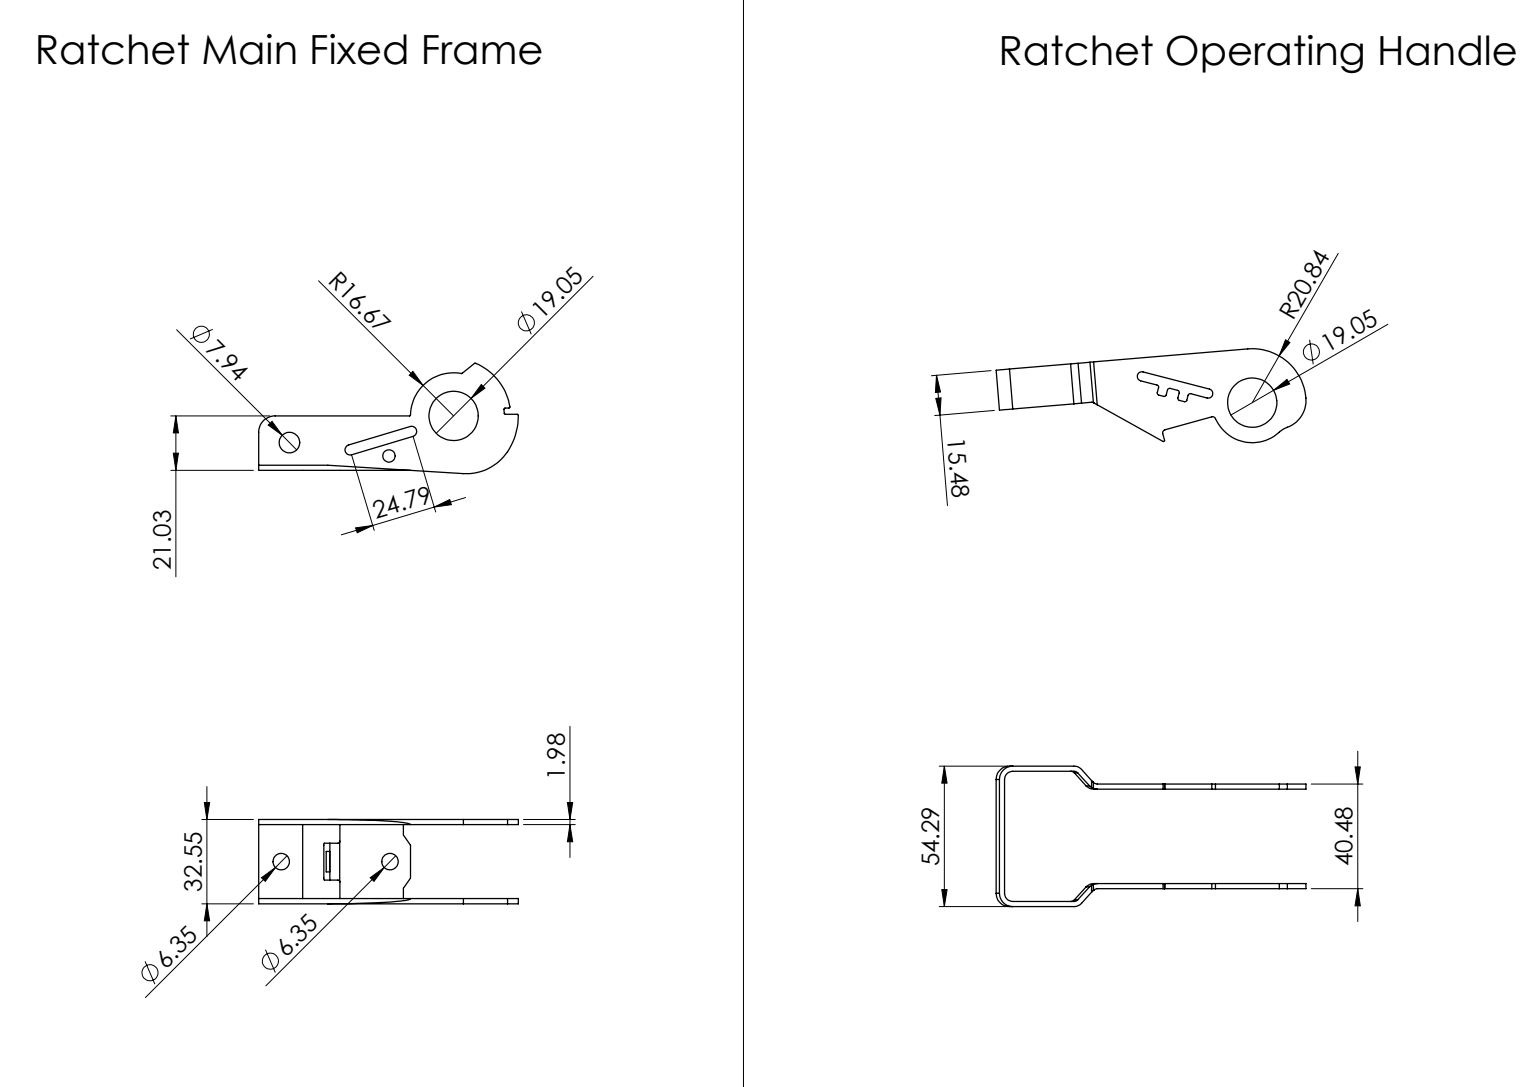
ISO-10303-21;
HEADER;
FILE_DESCRIPTION (('STEP AP214'),
    '1' );
FILE_NAME ('Ratchet Main Fixed Frame.step',
    '2026-10-09T14:10:49',
    ( '' ),
    ( '' ),
    'SwSTEP 2.0',
    'SolidWorks 2026',
    '' );
FILE_SCHEMA (( 'AUTOMOTIVE_DESIGN' ));
ENDSEC;

DATA;
#8=CARTESIAN_POINT ( 'NONE',  ( -23.01875000000000071, 1.984375000000000000, -3.968750000000000000 ) ) ;
#9=ADVANCED_FACE ( 'NONE', ( #16944, #16633 ), #1476, .F. ) ;
#15=CARTESIAN_POINT ( 'NONE',  ( -17.46249999999999858, 1.984375000000000000, 0.000000000000000000 ) ) ;
#18=CARTESIAN_POINT ( 'NONE',  ( 49.81956284419040060, 0.000000000000000000, 11.98436472153758103 ) ) ;
#22=VECTOR ( 'NONE', #6155, 999.9999999999998863 ) ;
#23=ORIENTED_EDGE ( 'NONE', *, *, #18650, .T. ) ;
#35=CARTESIAN_POINT ( 'NONE',  ( -29.36874999999999858, 2.380615000000000148, 8.335010000000000474 ) ) ;
#46=CIRCLE ( 'NONE', #17730, 1.984374999999999112 ) ;
#65=DIRECTION ( 'NONE',  ( 0.000000000000000000, 0.000000000000000000, -1.000000000000000000 ) ) ;
#67=AXIS2_PLACEMENT_3D ( 'NONE', #9052, #15829, #7402 ) ;
#70=ORIENTED_EDGE ( 'NONE', *, *, #12967, .F. ) ;
#71=AXIS2_PLACEMENT_3D ( 'NONE', #14766, #21802, #18271 ) ;
#74=PLANE ( 'NONE',  #18206 ) ;
#78=VECTOR ( 'NONE', #17853, 1000.000000000000227 ) ;
#94=AXIS2_PLACEMENT_3D ( 'NONE', #5064, #16687, #13274 ) ;
#104=CYLINDRICAL_SURFACE ( 'NONE', #7585, 0.3962400000000010358 ) ;
#109=CARTESIAN_POINT ( 'NONE',  ( 46.03750000000000142, 0.000000000000000000, -10.31874999999999964 ) ) ;
#117=CARTESIAN_POINT ( 'NONE',  ( 36.51250000000000284, 30.56064500000000095, -10.31875000000000142 ) ) ;
#120=EDGE_LOOP ( 'NONE', ( #10937, #5548, #3135, #2897 ) ) ;
#125=PLANE ( 'NONE',  #13958 ) ;
#133=DIRECTION ( 'NONE',  ( -0.9980811434661737147, 0.000000000000000000, -0.06191955310929838502 ) ) ;
#138=VERTEX_POINT ( 'NONE', #587 ) ;
#141=DIRECTION ( 'NONE',  ( 0.000000000000000000, 1.000000000000000000, 0.000000000000000000 ) ) ;
#150=DIRECTION ( 'NONE',  ( 0.000000000000000000, -1.000000000000000000, 0.000000000000000000 ) ) ;
#154=ORIENTED_EDGE ( 'NONE', *, *, #19245, .T. ) ;
#161=VECTOR ( 'NONE', #4886, 1000.000000000000227 ) ;
#162=LINE ( 'NONE', #18727, #15361 ) ;
#176=ORIENTED_EDGE ( 'NONE', *, *, #8308, .T. ) ;
#197=ORIENTED_EDGE ( 'NONE', *, *, #8367, .F. ) ;
#198=ORIENTED_EDGE ( 'NONE', *, *, #7883, .F. ) ;
#205=CARTESIAN_POINT ( 'NONE',  ( 29.36874999999999858, 0.000000000000000000, 10.71562499999999929 ) ) ;
#206=EDGE_LOOP ( 'NONE', ( #18423, #5151, #18532, #223 ) ) ;
#209=ORIENTED_EDGE ( 'NONE', *, *, #16573, .T. ) ;
#214=DIRECTION ( 'NONE',  ( 0.000000000000000000, 1.000000000000000000, 0.000000000000000000 ) ) ;
#218=VERTEX_POINT ( 'NONE', #12980 ) ;
#223=ORIENTED_EDGE ( 'NONE', *, *, #6828, .F. ) ;
#228=ORIENTED_EDGE ( 'NONE', *, *, #15345, .F. ) ;
#238=CARTESIAN_POINT ( 'NONE',  ( 54.11611804786240043, 30.56064500000000095, -30.58983753981140197 ) ) ;
#239=AXIS2_PLACEMENT_3D ( 'NONE', #18075, #4699, #2934 ) ;
#243=DIRECTION ( 'NONE',  ( -0.1831666983863990128, 0.000000000000000000, 0.9830818687180767901 ) ) ;
#259=LINE ( 'NONE', #5449, #10897 ) ;
#271=DIRECTION ( 'NONE',  ( 0.000000000000000000, 1.000000000000000000, 0.000000000000000000 ) ) ;
#280=DIRECTION ( 'NONE',  ( 0.000000000000000000, 1.000000000000000000, 0.000000000000000000 ) ) ;
#281=ORIENTED_EDGE ( 'NONE', *, *, #11678, .T. ) ;
#289=EDGE_CURVE ( 'NONE', #5674, #3944, #16188, .T. ) ;
#290=CARTESIAN_POINT ( 'NONE',  ( 6.016625000000000334, 1.984375000000000000, 2.794000000000000039 ) ) ;
#291=CARTESIAN_POINT ( 'NONE',  ( -29.36874999999999858, 9.129395000000000593, 0.000000000000000000 ) ) ;
#295=CARTESIAN_POINT ( 'NONE',  ( 18.65312499999999929, 0.000000000000000000, 5.159374999999999822 ) ) ;
#301=DIRECTION ( 'NONE',  ( 0.000000000000000000, 1.000000000000000000, 0.000000000000000000 ) ) ;
#311=EDGE_CURVE ( 'NONE', #1101, #20045, #18407, .T. ) ;
#313=DIRECTION ( 'NONE',  ( 0.000000000000000000, -1.000000000000000000, 0.000000000000000000 ) ) ;
#316=EDGE_CURVE ( 'NONE', #18861, #19124, #21090, .T. ) ;
#319=EDGE_CURVE ( 'NONE', #2537, #9809, #10285, .T. ) ;
#322=CARTESIAN_POINT ( 'NONE',  ( 1.954387715434429795, -42.42568807200000691, 6.745605000000000295 ) ) ;
#323=CARTESIAN_POINT ( 'NONE',  ( 67.40134256979101224, 0.000000000000000000, -13.70358117861468017 ) ) ;
#326=ORIENTED_EDGE ( 'NONE', *, *, #979, .T. ) ;
#354=DIRECTION ( 'NONE',  ( -0.9579671649362033747, 0.000000000000000000, 0.2868778675745011220 ) ) ;
#364=LINE ( 'NONE', #8871, #4198 ) ;
#377=VECTOR ( 'NONE', #1528, 1000.000000000000000 ) ;
#391=LINE ( 'NONE', #12123, #16283 ) ;
#395=VERTEX_POINT ( 'NONE', #5841 ) ;
#411=VECTOR ( 'NONE', #16269, 1000.000000000000114 ) ;
#417=ORIENTED_EDGE ( 'NONE', *, *, #10498, .T. ) ;
#418=EDGE_LOOP ( 'NONE', ( #15231, #7592, #4547, #16029 ) ) ;
#436=VECTOR ( 'NONE', #9326, 1000.000000000000000 ) ;
#442=DIRECTION ( 'NONE',  ( -0.2868778675745010664, 0.000000000000000000, -0.9579671649362032637 ) ) ;
#447=CARTESIAN_POINT ( 'NONE',  ( -29.36874999999999858, 0.000000000000000000, -3.968750000000000000 ) ) ;
#468=EDGE_CURVE ( 'NONE', #14260, #16212, #12495, .T. ) ;
#501=EDGE_LOOP ( 'NONE', ( #16352, #7920, #20206, #7975 ) ) ;
#505=ORIENTED_EDGE ( 'NONE', *, *, #10172, .T. ) ;
#507=DIRECTION ( 'NONE',  ( 0.000000000000000000, -1.000000000000000000, 0.000000000000000000 ) ) ;
#511=ORIENTED_EDGE ( 'NONE', *, *, #13513, .F. ) ;
#516=ORIENTED_EDGE ( 'NONE', *, *, #17729, .F. ) ;
#518=AXIS2_PLACEMENT_3D ( 'NONE', #7879, #21361, #11096 ) ;
#528=CARTESIAN_POINT ( 'NONE',  ( 46.03750000000000142, 0.000000000000000000, -10.31874999999999964 ) ) ;
#554=CIRCLE ( 'NONE', #4091, 0.3962399999999999811 ) ;
#564=EDGE_LOOP ( 'NONE', ( #7716, #9815, #9669, #1208 ) ) ;
#572=PLANE ( 'NONE',  #16036 ) ;
#581=CARTESIAN_POINT ( 'NONE',  ( 29.19635173153840313, 32.54502000000000095, -6.218966092919240296 ) ) ;
#582=FACE_BOUND ( 'NONE', #7037, .T. ) ;
#587=CARTESIAN_POINT ( 'NONE',  ( 49.41235866845560309, 32.54502000000000095, -26.78690084448080100 ) ) ;
#622=CARTESIAN_POINT ( 'NONE',  ( 65.90927232300019512, 0.000000000000000000, -13.30734117861468135 ) ) ;
#628=ORIENTED_EDGE ( 'NONE', *, *, #11808, .F. ) ;
#629=CYLINDRICAL_SURFACE ( 'NONE', #3313, 0.3962399999999990929 ) ;
#630=CARTESIAN_POINT ( 'NONE',  ( 1.952969610814715207, 8.739187247087119914, 8.731249999999999289 ) ) ;
#632=ORIENTED_EDGE ( 'NONE', *, *, #7507, .T. ) ;
#641=EDGE_CURVE ( 'NONE', #1856, #20988, #8151, .T. ) ;
#642=ORIENTED_EDGE ( 'NONE', *, *, #17287, .T. ) ;
#646=CARTESIAN_POINT ( 'NONE',  ( 18.74375446079810104, 0.5063334429457699848, 10.05646519131946093 ) ) ;
#648=DIRECTION ( 'NONE',  ( 0.000000000000000000, -1.000000000000000000, 0.000000000000000000 ) ) ;
#655=DIRECTION ( 'NONE',  ( 0.000000000000000000, 1.000000000000000000, 0.000000000000000000 ) ) ;
#656=DIRECTION ( 'NONE',  ( 0.000000000000000000, -1.000000000000000000, 0.000000000000000000 ) ) ;
#658=ORIENTED_EDGE ( 'NONE', *, *, #14396, .F. ) ;
#664=EDGE_LOOP ( 'NONE', ( #18136, #17984, #7800, #6958 ) ) ;
#665=EDGE_CURVE ( 'NONE', #14162, #4933, #12805, .T. ) ;
#677=CYLINDRICAL_SURFACE ( 'NONE', #11422, 0.3962400000000008138 ) ;
#691=EDGE_CURVE ( 'NONE', #3431, #18275, #1843, .T. ) ;
#695=ORIENTED_EDGE ( 'NONE', *, *, #7242, .F. ) ;
#705=EDGE_CURVE ( 'NONE', #1101, #3875, #6823, .T. ) ;
#708=LINE ( 'NONE', #15884, #14164 ) ;
#710=EDGE_LOOP ( 'NONE', ( #9718, #14667, #1796, #5850, #15920 ) ) ;
#717=LINE ( 'NONE', #12670, #3287 ) ;
#726=CARTESIAN_POINT ( 'NONE',  ( 1.268730000000000135, 9.129395000000000593, 8.609509071587499562 ) ) ;
#729=CIRCLE ( 'NONE', #7799, 2.381250000000001421 ) ;
#731=EDGE_LOOP ( 'NONE', ( #7711, #2068 ) ) ;
#733=AXIS2_PLACEMENT_3D ( 'NONE', #2522, #9471, #14263 ) ;
#735=EDGE_CURVE ( 'NONE', #12688, #16536, #11693, .T. ) ;
#738=LINE ( 'NONE', #19310, #21439 ) ;
#739=VECTOR ( 'NONE', #11879, 1000.000000000000000 ) ;
#743=ADVANCED_FACE ( 'NONE', ( #9913 ), #18750, .T. ) ;
#757=CARTESIAN_POINT ( 'NONE',  ( 6.472296726610020201, 0.08030987734106199982, 9.295161179239141092 ) ) ;
#764=EDGE_CURVE ( 'NONE', #7013, #13795, #15358, .T. ) ;
#765=ORIENTED_EDGE ( 'NONE', *, *, #8954, .T. ) ;
#768=DIRECTION ( 'NONE',  ( 0.2868778675745004558, 0.000000000000000000, 0.9579671649362035968 ) ) ;
#771=EDGE_LOOP ( 'NONE', ( #6023, #8487, #4066, #14596 ) ) ;
#772=ORIENTED_EDGE ( 'NONE', *, *, #5768, .T. ) ;
#777=VERTEX_POINT ( 'NONE', #19975 ) ;
#793=VECTOR ( 'NONE', #3732, 1000.000000000000114 ) ;
#796=DIRECTION ( 'NONE',  ( 0.000000000000000000, 1.000000000000000000, 0.000000000000000000 ) ) ;
#798=CARTESIAN_POINT ( 'NONE',  ( 6.585898268469219552, 30.56064500000000095, 4.694966092919240275 ) ) ;
#812=DIRECTION ( 'NONE',  ( 0.000000000000000000, 1.000000000000000000, 0.000000000000000000 ) ) ;
#817=AXIS2_PLACEMENT_3D ( 'NONE', #3190, #18327, #3407 ) ;
#818=CARTESIAN_POINT ( 'NONE',  ( -2.028188046367890074, 9.924415000000001541, 0.3682158094503220069 ) ) ;
#825=VECTOR ( 'NONE', #16124, 1000.000000000000227 ) ;
#827=DIRECTION ( 'NONE',  ( 0.000000000000000000, 1.000000000000000000, 0.000000000000000000 ) ) ;
#833=CARTESIAN_POINT ( 'NONE',  ( 26.59062499999999929, 2.380615000000000148, 8.731249999999999289 ) ) ;
#840=CARTESIAN_POINT ( 'NONE',  ( 26.59062499999999929, 5.953125000000000000, 10.71562499999999929 ) ) ;
#843=EDGE_CURVE ( 'NONE', #5953, #16263, #20185, .T. ) ;
#852=CIRCLE ( 'NONE', #12513, 0.3962399999999990929 ) ;
#854=EDGE_LOOP ( 'NONE', ( #772, #16081, #18567, #4619, #13382, #13035, #9205, #19390, #3885, #9519, #20998, #18124, #9666, #2739, #11741, #2851, #8488, #10820, #3221, #4979, #18354 ) ) ;
#857=AXIS2_PLACEMENT_3D ( 'NONE', #12113, #15668, #1410 ) ;
#860=FACE_OUTER_BOUND ( 'NONE', #15123, .T. ) ;
#873=CARTESIAN_POINT ( 'NONE',  ( 11.57071721368057915, 0.2046444788096904999, 9.611460029477360223 ) ) ;
#894=DIRECTION ( 'NONE',  ( 0.2868778675745010664, 0.000000000000000000, 0.9579671649362032637 ) ) ;
#896=EDGE_CURVE ( 'NONE', #10916, #13402, #20547, .T. ) ;
#908=CARTESIAN_POINT ( 'NONE',  ( 1.336191582698512681, 23.41816499999998769, 10.66779613908654056 ) ) ;
#915=CARTESIAN_POINT ( 'NONE',  ( 29.35287372532640049, 1.909660849011530104, 10.71464187463071838 ) ) ;
#922=ADVANCED_FACE ( 'NONE', ( #2286 ), #10909, .F. ) ;
#937=DIRECTION ( 'NONE',  ( 0.000000000000000000, 0.000000000000000000, 1.000000000000000000 ) ) ;
#943=EDGE_CURVE ( 'NONE', #17008, #1261, #5484, .T. ) ;
#955=DIRECTION ( 'NONE',  ( 1.000000000000000000, 0.000000000000000000, 0.000000000000000000 ) ) ;
#958=CARTESIAN_POINT ( 'NONE',  ( 65.90927232300019512, 32.54502000000000095, -13.30734117861468135 ) ) ;
#966=VERTEX_POINT ( 'NONE', #17658 ) ;
#971=CARTESIAN_POINT ( 'NONE',  ( 2.063750000000000195, 1.984375000000000000, -16.49278420930464861 ) ) ;
#974=ORIENTED_EDGE ( 'NONE', *, *, #1086, .T. ) ;
#978=CARTESIAN_POINT ( 'NONE',  ( -29.36874999999999858, 2.380615000000000148, 8.731249999999999289 ) ) ;
#979=EDGE_CURVE ( 'NONE', #12825, #9462, #12474, .T. ) ;
#986=ORIENTED_EDGE ( 'NONE', *, *, #17962, .F. ) ;
#1004=CARTESIAN_POINT ( 'NONE',  ( 2.063750000000000195, 24.21318500000000284, 10.71562499999999929 ) ) ;
#1007=DIRECTION ( 'NONE',  ( 1.000000000000000000, 0.000000000000000000, 0.000000000000000000 ) ) ;
#1012=PRODUCT_DEFINITION ( 'UNKNOWN', '', #20389, #10115 ) ;
#1016=CARTESIAN_POINT ( 'NONE',  ( 26.96090640492720425, 1.228048945539309766, 10.56624576331076071 ) ) ;
#1019=DIRECTION ( 'NONE',  ( -0.9966381950048638361, 0.000000000000000000, 0.08192867786951606168 ) ) ;
#1025=ORIENTED_EDGE ( 'NONE', *, *, #19522, .F. ) ;
#1027=DIRECTION ( 'NONE',  ( 1.000000000000000000, 0.000000000000000000, 0.000000000000000000 ) ) ;
#1031=FACE_OUTER_BOUND ( 'NONE', #17461, .T. ) ;
#1040=ORIENTED_EDGE ( 'NONE', *, *, #6973, .F. ) ;
#1051=CIRCLE ( 'NONE', #4594, 0.3962399999999999811 ) ;
#1058=( GEOMETRIC_REPRESENTATION_CONTEXT ( 3 ) GLOBAL_UNCERTAINTY_ASSIGNED_CONTEXT ( ( #18944 ) ) GLOBAL_UNIT_ASSIGNED_CONTEXT ( ( #20231, #6550, #3348 ) ) REPRESENTATION_CONTEXT ( 'NONE', 'WORKASPACE' ) );
#1061=CARTESIAN_POINT ( 'NONE',  ( 70.64340948846358970, 32.54502000000000095, -10.93409647675949969 ) ) ;
#1062=ORIENTED_EDGE ( 'NONE', *, *, #13513, .T. ) ;
#1067=ORIENTED_EDGE ( 'NONE', *, *, #1108, .F. ) ;
#1076=ORIENTED_EDGE ( 'NONE', *, *, #468, .T. ) ;
#1082=AXIS2_PLACEMENT_3D ( 'NONE', #19728, #13446, #18513 ) ;
#1084=CARTESIAN_POINT ( 'NONE',  ( 46.03750000000000142, 32.54502000000000095, -10.31874999999999964 ) ) ;
#1086=EDGE_CURVE ( 'NONE', #10374, #6204, #17753, .T. ) ;
#1087=AXIS2_PLACEMENT_3D ( 'NONE', #11496, #6526, #8379 ) ;
#1094=FACE_OUTER_BOUND ( 'NONE', #16465, .T. ) ;
#1101=VERTEX_POINT ( 'NONE', #21702 ) ;
#1107=AXIS2_PLACEMENT_3D ( 'NONE', #8605, #15486, #8489 ) ;
#1108=EDGE_CURVE ( 'NONE', #9462, #16780, #13415, .T. ) ;
#1111=DIRECTION ( 'NONE',  ( -0.9579671649362032637, 0.000000000000000000, 0.2868778675745010664 ) ) ;
#1120=DIRECTION ( 'NONE',  ( 0.000000000000000000, 0.000000000000000000, 1.000000000000000000 ) ) ;
#1127=CARTESIAN_POINT ( 'NONE',  ( 28.31895198753520049, 1.479004908355108006, 10.65049700491969986 ) ) ;
#1132=DIRECTION ( 'NONE',  ( 1.000000000000000000, 0.000000000000000000, 0.000000000000000000 ) ) ;
#1135=DIRECTION ( 'NONE',  ( 0.000000000000000000, 1.000000000000000000, 0.000000000000000000 ) ) ;
#1139=AXIS2_PLACEMENT_3D ( 'NONE', #15940, #16049, #10935 ) ;
#1140=CYLINDRICAL_SURFACE ( 'NONE', #6685, 22.02656249999999361 ) ;
#1142=CARTESIAN_POINT ( 'NONE',  ( 6.016625000000000334, 32.54502000000000095, 2.794000000000000039 ) ) ;
#1145=CIRCLE ( 'NONE', #3270, 6.349999999999999645 ) ;
#1156=VECTOR ( 'NONE', #3402, 1000.000000000000000 ) ;
#1161=DIRECTION ( 'NONE',  ( 0.000000000000000000, 1.000000000000000000, 0.000000000000000000 ) ) ;
#1162=ORIENTED_EDGE ( 'NONE', *, *, #15592, .F. ) ;
#1164=EDGE_LOOP ( 'NONE', ( #7263, #18315, #20283, #12931 ) ) ;
#1168=ADVANCED_FACE ( 'NONE', ( #11530 ), #8094, .T. ) ;
#1171=ORIENTED_EDGE ( 'NONE', *, *, #15592, .T. ) ;
#1179=ORIENTED_EDGE ( 'NONE', *, *, #6973, .T. ) ;
#1182=ORIENTED_EDGE ( 'NONE', *, *, #6183, .F. ) ;
#1186=DIRECTION ( 'NONE',  ( 0.000000000000000000, -1.000000000000000000, 0.000000000000000000 ) ) ;
#1187=EDGE_LOOP ( 'NONE', ( #19885, #4119, #17539, #10765 ) ) ;
#1195=VECTOR ( 'NONE', #7827, 999.9999999999998863 ) ;
#1202=VERTEX_POINT ( 'NONE', #19816 ) ;
#1204=CARTESIAN_POINT ( 'NONE',  ( 26.59062499871549790, 1.984216250000009785, 10.71562498306123956 ) ) ;
#1208=ORIENTED_EDGE ( 'NONE', *, *, #20286, .F. ) ;
#1212=DIRECTION ( 'NONE',  ( 1.000000000000000000, 0.000000000000000000, 0.000000000000000000 ) ) ;
#1215=EDGE_LOOP ( 'NONE', ( #5293, #9550, #511, #6847 ) ) ;
#1239=DIRECTION ( 'NONE',  ( -0.7776383362760926898, 0.000000000000000000, 0.6287118719681938916 ) ) ;
#1243=DIRECTION ( 'NONE',  ( 1.000000000000000000, 0.000000000000000000, 0.000000000000000000 ) ) ;
#1249=DIRECTION ( 'NONE',  ( 0.000000000000000000, 1.000000000000000000, 0.000000000000000000 ) ) ;
#1252=CARTESIAN_POINT ( 'NONE',  ( -3.929154139288399961, 22.62314500000000095, 0.9374890779182719625 ) ) ;
#1256=EDGE_LOOP ( 'NONE', ( #8055, #5991, #15134, #11048, #17890, #4299 ) ) ;
#1260=AXIS2_PLACEMENT_3D ( 'NONE', #13322, #14664, #16739 ) ;
#1261=VERTEX_POINT ( 'NONE', #10524 ) ;
#1266=VERTEX_POINT ( 'NONE', #12086 ) ;
#1286=CARTESIAN_POINT ( 'NONE',  ( 21.03437500000000071, 30.56064500000000095, 5.159374999999999822 ) ) ;
#1302=CARTESIAN_POINT ( 'NONE',  ( 71.03963378001139972, 32.54502000000000095, -10.54138470677948014 ) ) ;
#1307=CARTESIAN_POINT ( 'NONE',  ( 201.9384738932629944, 1.984375000000000000, 10.71562489836746046 ) ) ;
#1311=EDGE_CURVE ( 'NONE', #7810, #19275, #7545, .T. ) ;
#1319=DIRECTION ( 'NONE',  ( 0.2868778675745004558, 0.000000000000000000, 0.9579671649362035968 ) ) ;
#1331=CARTESIAN_POINT ( 'NONE',  ( 1.603561069792159621, 23.48871702854725996, 10.70056859876313382 ) ) ;
#1335=ORIENTED_EDGE ( 'NONE', *, *, #3563, .F. ) ;
#1344=FACE_OUTER_BOUND ( 'NONE', #19634, .T. ) ;
#1346=DIRECTION ( 'NONE',  ( 0.000000000000000000, -1.000000000000000000, 0.000000000000000000 ) ) ;
#1349=AXIS2_PLACEMENT_3D ( 'NONE', #35, #13658, #3583 ) ;
#1356=VERTEX_POINT ( 'NONE', #2346 ) ;
#1378=CIRCLE ( 'NONE', #4216, 0.3962399999999988154 ) ;
#1385=ADVANCED_FACE ( 'NONE', ( #4114 ), #10856, .F. ) ;
#1386=ADVANCED_FACE ( 'NONE', ( #17394 ), #7323, .T. ) ;
#1389=CARTESIAN_POINT ( 'NONE',  ( 46.03750000000000142, 0.000000000000000000, -10.31874999999999964 ) ) ;
#1394=CARTESIAN_POINT ( 'NONE',  ( 55.56250000000000000, 30.56064500000000095, -10.31874999999999964 ) ) ;
#1395=ORIENTED_EDGE ( 'NONE', *, *, #4129, .T. ) ;
#1399=ORIENTED_EDGE ( 'NONE', *, *, #12967, .T. ) ;
#1402=VERTEX_POINT ( 'NONE', #798 ) ;
#1410=DIRECTION ( 'NONE',  ( 1.000000000000000000, 0.000000000000000000, 0.000000000000000000 ) ) ;
#1413=EDGE_CURVE ( 'NONE', #10320, #7268, #19359, .T. ) ;
#1417=CARTESIAN_POINT ( 'NONE',  ( 46.03750000000000142, 30.56064500000000095, -10.31874999999999964 ) ) ;
#1418=FACE_OUTER_BOUND ( 'NONE', #9038, .T. ) ;
#1420=ORIENTED_EDGE ( 'NONE', *, *, #5878, .F. ) ;
#1421=ORIENTED_EDGE ( 'NONE', *, *, #14670, .T. ) ;
#1424=CARTESIAN_POINT ( 'NONE',  ( 67.40134256979101224, 32.54502000000000095, -13.30734117861468135 ) ) ;
#1427=CARTESIAN_POINT ( 'NONE',  ( 26.59062499999999929, 5.953125000000000000, 8.731249999999999289 ) ) ;
#1428=AXIS2_PLACEMENT_3D ( 'NONE', #20915, #20685, #5542 ) ;
#1432=EDGE_CURVE ( 'NONE', #6164, #7181, #16178, .T. ) ;
#1433=VECTOR ( 'NONE', #5276, 1000.000000000000000 ) ;
#1441=DIRECTION ( 'NONE',  ( 0.9966381950048638361, 0.000000000000000000, -0.08192867786951699149 ) ) ;
#1445=EDGE_LOOP ( 'NONE', ( #18109, #19711, #10943, #9247 ) ) ;
#1449=VERTEX_POINT ( 'NONE', #21235 ) ;
#1451=VECTOR ( 'NONE', #4832, 1000.000000000000000 ) ;
#1453=LINE ( 'NONE', #21355, #13072 ) ;
#1455=AXIS2_PLACEMENT_3D ( 'NONE', #16323, #11654, #19616 ) ;
#1458=DIRECTION ( 'NONE',  ( 0.2868778675745011220, 0.000000000000000000, 0.9579671649362033747 ) ) ;
#1469=CARTESIAN_POINT ( 'NONE',  ( -2.256261688646920227, 9.924415000000001541, -0.3933872460174320240 ) ) ;
#1476=PLANE ( 'NONE',  #5340 ) ;
#1486=DIRECTION ( 'NONE',  ( -0.9579671649362032637, 0.000000000000000000, 0.2868778675745010664 ) ) ;
#1498=FACE_OUTER_BOUND ( 'NONE', #6214, .T. ) ;
#1502=CARTESIAN_POINT ( 'NONE',  ( 65.64431122251959039, 0.000000000000000000, -11.29787305743958115 ) ) ;
#1503=EDGE_LOOP ( 'NONE', ( #2825, #2613, #15196, #20000 ) ) ;
#1522=CARTESIAN_POINT ( 'NONE',  ( 54.11611804786240043, 1.984375000000000000, -30.58983753981140197 ) ) ;
#1523=DIRECTION ( 'NONE',  ( 0.000000000000000000, 0.000000000000000000, -1.000000000000000000 ) ) ;
#1528=DIRECTION ( 'NONE',  ( 0.000000000000000000, 1.000000000000000000, 0.000000000000000000 ) ) ;
#1534=DIRECTION ( 'NONE',  ( 1.000000000000000000, 0.000000000000000000, 0.000000000000000000 ) ) ;
#1539=CARTESIAN_POINT ( 'NONE',  ( -12.30312499999999964, 30.56064500000000095, 8.731249999999999289 ) ) ;
#1543=EDGE_CURVE ( 'NONE', #10050, #7714, #3297, .T. ) ;
#1547=PLANE ( 'NONE',  #20270 ) ;
#1550=ORIENTED_EDGE ( 'NONE', *, *, #5921, .F. ) ;
#1552=AXIS2_PLACEMENT_3D ( 'NONE', #9619, #13292, #21231 ) ;
#1553=PLANE ( 'NONE',  #6412 ) ;
#1561=EDGE_CURVE ( 'NONE', #16780, #6164, #2753, .T. ) ;
#1572=DIRECTION ( 'NONE',  ( -0.7776383362760926898, 0.000000000000000000, 0.6287118719681938916 ) ) ;
#1576=DIRECTION ( 'NONE',  ( 0.000000000000000000, 1.000000000000000000, 0.000000000000000000 ) ) ;
#1589=CARTESIAN_POINT ( 'NONE',  ( 26.59062499999999929, 2.380615000000000148, 8.335010000000000474 ) ) ;
#1593=CARTESIAN_POINT ( 'NONE',  ( -29.36874999999999858, 30.16440499999999858, 8.731249999999999289 ) ) ;
#1626=EDGE_LOOP ( 'NONE', ( #16316, #15503, #7681, #7730 ) ) ;
#1629=CARTESIAN_POINT ( 'NONE',  ( 46.03750000000000142, 1.984375000000000000, -10.31874999999999964 ) ) ;
#1639=LINE ( 'NONE', #3320, #14876 ) ;
#1641=ORIENTED_EDGE ( 'NONE', *, *, #12188, .F. ) ;
#1644=EDGE_CURVE ( 'NONE', #11015, #3875, #17773, .T. ) ;
#1648=CARTESIAN_POINT ( 'NONE',  ( -4.157227781567939928, 9.129395000000000593, 0.1758860224507720060 ) ) ;
#1655=CARTESIAN_POINT ( 'NONE',  ( -17.46249999999999858, 30.56064500000000095, 0.000000000000000000 ) ) ;
#1659=ADVANCED_FACE ( 'NONE', ( #17113 ), #3627, .F. ) ;
#1668=CARTESIAN_POINT ( 'NONE',  ( 54.29867169743560140, 0.000000000000000000, -30.73743011777780154 ) ) ;
#1672=CARTESIAN_POINT ( 'NONE',  ( 28.97711086133420366, 32.54502000000000095, -10.71499000000000024 ) ) ;
#1683=DIRECTION ( 'NONE',  ( 0.000000000000000000, 1.000000000000000000, 0.000000000000000000 ) ) ;
#1684=DIRECTION ( 'NONE',  ( 1.000000000000000000, 0.000000000000000000, 0.000000000000000000 ) ) ;
#1686=CARTESIAN_POINT ( 'NONE',  ( 5.447351731530780228, 30.56064500000000095, 0.8930339070797439494 ) ) ;
#1694=CARTESIAN_POINT ( 'NONE',  ( 46.03750000000000142, 0.000000000000000000, -10.31874999999999964 ) ) ;
#1704=EDGE_CURVE ( 'NONE', #17862, #13475, #2935, .T. ) ;
#1709=ORIENTED_EDGE ( 'NONE', *, *, #4496, .T. ) ;
#1713=B_SPLINE_CURVE_WITH_KNOTS ( 'NONE', 3,
 ( #12498, #7513, #19221, #4190, #10495, #15718, #17682, #2534 ),
 .UNSPECIFIED., .F., .F.,
 ( 4, 2, 2, 4 ),
 ( 0.000000000000000000, 0.2499999999999987232, 0.4999999999999974465, 1.000000000000000000 ),
 .UNSPECIFIED. ) ;
#1714=VERTEX_POINT ( 'NONE', #6609 ) ;
#1728=AXIS2_PLACEMENT_3D ( 'NONE', #5068, #1959, #20517 ) ;
#1734=VECTOR ( 'NONE', #18310, 1000.000000000000114 ) ;
#1736=DIRECTION ( 'NONE',  ( 0.000000000000000000, 1.000000000000000000, 0.000000000000000000 ) ) ;
#1737=CARTESIAN_POINT ( 'NONE',  ( 46.03750000000000142, 32.54502000000000095, -10.31874999999999964 ) ) ;
#1739=LINE ( 'NONE', #5067, #13841 ) ;
#1747=ORIENTED_EDGE ( 'NONE', *, *, #6828, .T. ) ;
#1748=DIRECTION ( 'NONE',  ( 0.000000000000000000, 1.000000000000000000, 0.000000000000000000 ) ) ;
#1751=EDGE_CURVE ( 'NONE', #4180, #17367, #17419, .T. ) ;
#1752=DIRECTION ( 'NONE',  ( 0.9999603561554373243, 0.000000000000000000, -0.008904275236710241376 ) ) ;
#1753=CARTESIAN_POINT ( 'NONE',  ( 29.37324403177899868, 0.000000000000000000, -10.70578951775076071 ) ) ;
#1756=FACE_OUTER_BOUND ( 'NONE', #854, .T. ) ;
#1771=DIRECTION ( 'NONE',  ( 0.000000000000000000, 1.000000000000000000, 0.000000000000000000 ) ) ;
#1774=AXIS2_PLACEMENT_3D ( 'NONE', #10053, #8282, #6290 ) ;
#1776=FACE_OUTER_BOUND ( 'NONE', #9027, .T. ) ;
#1796=ORIENTED_EDGE ( 'NONE', *, *, #10074, .F. ) ;
#1798=CARTESIAN_POINT ( 'NONE',  ( 71.04062499999999147, 0.000000000000000000, -10.31874999999999964 ) ) ;
#1801=ORIENTED_EDGE ( 'NONE', *, *, #20190, .T. ) ;
#1825=CIRCLE ( 'NONE', #3243, 1.984374999999998890 ) ;
#1831=ORIENTED_EDGE ( 'NONE', *, *, #17908, .T. ) ;
#1838=ORIENTED_EDGE ( 'NONE', *, *, #10629, .F. ) ;
#1839=DIRECTION ( 'NONE',  ( 0.000000000000000000, 1.000000000000000000, 0.000000000000000000 ) ) ;
#1843=LINE ( 'NONE', #15037, #8191 ) ;
#1856=VERTEX_POINT ( 'NONE', #19308 ) ;
#1859=CARTESIAN_POINT ( 'NONE',  ( -29.36874999999999858, 0.000000000000000000, 8.731885000000000119 ) ) ;
#1871=ORIENTED_EDGE ( 'NONE', *, *, #10172, .F. ) ;
#1876=VERTEX_POINT ( 'NONE', #4170 ) ;
#1882=ORIENTED_EDGE ( 'NONE', *, *, #3188, .T. ) ;
#1891=EDGE_CURVE ( 'NONE', #21568, #12583, #7167, .T. ) ;
#1893=CIRCLE ( 'NONE', #8262, 3.175000000000000711 ) ;
#1895=CARTESIAN_POINT ( 'NONE',  ( -20.63749999999999929, 16.27314499999999953, 8.731249999999999289 ) ) ;
#1898=DIRECTION ( 'NONE',  ( 0.000000000000000000, -1.000000000000000000, 0.000000000000000000 ) ) ;
#1900=AXIS2_PLACEMENT_3D ( 'NONE', #18001, #14482, #6058 ) ;
#1908=CARTESIAN_POINT ( 'NONE',  ( 6.585898268469219552, 1.984375000000000000, 4.694966092919240275 ) ) ;
#1917=ORIENTED_EDGE ( 'NONE', *, *, #6375, .F. ) ;
#1931=ORIENTED_EDGE ( 'NONE', *, *, #21706, .T. ) ;
#1954=ORIENTED_EDGE ( 'NONE', *, *, #11915, .F. ) ;
#1958=CARTESIAN_POINT ( 'NONE',  ( 26.59062499999999929, 2.380615000000000148, 8.731249999999999289 ) ) ;
#1959=DIRECTION ( 'NONE',  ( 0.000000000000000000, 1.000000000000000000, 0.000000000000000000 ) ) ;
#1972=LINE ( 'NONE', #15490, #17384 ) ;
#1975=ADVANCED_FACE ( 'NONE', ( #3738 ), #629, .F. ) ;
#1977=DIRECTION ( 'NONE',  ( 0.000000000000000000, 0.000000000000000000, -1.000000000000000000 ) ) ;
#2020=VERTEX_POINT ( 'NONE', #20740 ) ;
#2027=DIRECTION ( 'NONE',  ( 1.000000000000000000, 0.000000000000000000, 0.000000000000000000 ) ) ;
#2032=ORIENTED_EDGE ( 'NONE', *, *, #19528, .F. ) ;
#2034=DIRECTION ( 'NONE',  ( 0.000000000000000000, -1.000000000000000000, 0.000000000000000000 ) ) ;
#2047=EDGE_CURVE ( 'NONE', #18768, #2822, #14695, .T. ) ;
#2051=CARTESIAN_POINT ( 'NONE',  ( -29.36874999999999858, 30.56128000000000000, 10.71562499999999929 ) ) ;
#2053=CARTESIAN_POINT ( 'NONE',  ( 0.02083138522551555155, 12.30439499999999953, 7.210477125664100484 ) ) ;
#2055=CARTESIAN_POINT ( 'NONE',  ( 1.402240371799016394, 9.120973559619994120, 10.67764259629631951 ) ) ;
#2063=ORIENTED_EDGE ( 'NONE', *, *, #15564, .F. ) ;
#2068=ORIENTED_EDGE ( 'NONE', *, *, #11302, .T. ) ;
#2076=CIRCLE ( 'NONE', #7372, 3.968750000000000000 ) ;
#2079=DIRECTION ( 'NONE',  ( 0.000000000000000000, 0.000000000000000000, -1.000000000000000000 ) ) ;
#2081=CARTESIAN_POINT ( 'NONE',  ( 17.77223365658175069, 0.4543760498246959822, 9.996193404372801794 ) ) ;
#2082=CIRCLE ( 'NONE', #15531, 0.7950200000000000600 ) ;
#2087=LINE ( 'NONE', #20216, #11922 ) ;
#2089=CARTESIAN_POINT ( 'NONE',  ( -3.246390552019219999, 12.30439499999999953, 3.217431771123079987 ) ) ;
#2091=LINE ( 'NONE', #10831, #6773 ) ;
#2092=ORIENTED_EDGE ( 'NONE', *, *, #11972, .F. ) ;
#2108=EDGE_CURVE ( 'NONE', #10320, #2958, #18819, .T. ) ;
#2113=DIRECTION ( 'NONE',  ( 0.000000000000000000, 1.000000000000000000, 0.000000000000000000 ) ) ;
#2122=VECTOR ( 'NONE', #827, 1000.000000000000000 ) ;
#2127=AXIS2_PLACEMENT_3D ( 'NONE', #12879, #11421, #1243 ) ;
#2137=ORIENTED_EDGE ( 'NONE', *, *, #16907, .F. ) ;
#2146=CARTESIAN_POINT ( 'NONE',  ( 65.51436440461340283, 0.000000000000000000, -12.87863775929475985 ) ) ;
#2151=EDGE_LOOP ( 'NONE', ( #4488, #19389, #2830, #5520 ) ) ;
#2159=CIRCLE ( 'NONE', #15957, 0.7950199999999998379 ) ;
#2165=CIRCLE ( 'NONE', #14549, 1.983739999999999393 ) ;
#2167=ORIENTED_EDGE ( 'NONE', *, *, #18913, .F. ) ;
#2173=CARTESIAN_POINT ( 'NONE',  ( 1.603642987080700744, 9.058787236897966721, 10.70057449157679663 ) ) ;
#2178=CARTESIAN_POINT ( 'NONE',  ( 71.03963378001139972, 0.000000000000000000, -10.54138470677948014 ) ) ;
#2179=CARTESIAN_POINT ( 'NONE',  ( 26.59062499999999929, 30.56064500000000095, 8.335010000000000474 ) ) ;
#2212=VERTEX_POINT ( 'NONE', #17883 ) ;
#2217=VERTEX_POINT ( 'NONE', #21294 ) ;
#2219=DIRECTION ( 'NONE',  ( 0.000000000000000000, 1.000000000000000000, 0.000000000000000000 ) ) ;
#2221=CIRCLE ( 'NONE', #3289, 0.3962399999999997591 ) ;
#2226=CARTESIAN_POINT ( 'NONE',  ( 1.954387715434429795, 8.736780638212259475, 10.71562499999999929 ) ) ;
#2228=ADVANCED_FACE ( 'NONE', ( #5563 ), #3924, .T. ) ;
#2234=AXIS2_PLACEMENT_3D ( 'NONE', #14022, #2275, #17644 ) ;
#2236=CYLINDRICAL_SURFACE ( 'NONE', #1428, 0.7950200000000000600 ) ;
#2237=CARTESIAN_POINT ( 'NONE',  ( -2.256261688646920227, 9.129395000000000593, -0.3933872460174320240 ) ) ;
#2240=EDGE_CURVE ( 'NONE', #20891, #13567, #9292, .T. ) ;
#2243=ORIENTED_EDGE ( 'NONE', *, *, #1751, .F. ) ;
#2247=DIRECTION ( 'NONE',  ( 0.9579671649362032637, 0.000000000000000000, -0.2868778675745010664 ) ) ;
#2262=EDGE_CURVE ( 'NONE', #2328, #20984, #4718, .T. ) ;
#2273=DIRECTION ( 'NONE',  ( 0.000000000000000000, 0.000000000000000000, -1.000000000000000000 ) ) ;
#2275=DIRECTION ( 'NONE',  ( 0.000000000000000000, 0.000000000000000000, 1.000000000000000000 ) ) ;
#2286=FACE_OUTER_BOUND ( 'NONE', #4386, .T. ) ;
#2293=FACE_OUTER_BOUND ( 'NONE', #15401, .T. ) ;
#2294=CARTESIAN_POINT ( 'NONE',  ( -1.880134707694870011, 20.24316500000000119, 7.779750394130780400 ) ) ;
#2307=CARTESIAN_POINT ( 'NONE',  ( -0.02450470937351344886, 0.004533752046478279826, 8.892108737872939983 ) ) ;
#2325=DIRECTION ( 'NONE',  ( 0.000000000000000000, 1.000000000000000000, 0.000000000000000000 ) ) ;
#2327=EDGE_LOOP ( 'NONE', ( #10719, #6356, #8378, #18238 ) ) ;
#2328=VERTEX_POINT ( 'NONE', #9649 ) ;
#2336=EDGE_CURVE ( 'NONE', #15924, #15199, #7891, .T. ) ;
#2340=DIRECTION ( 'NONE',  ( 0.9876802608827760510, 0.000000000000000000, -0.1564854698127960131 ) ) ;
#2343=ADVANCED_FACE ( 'NONE', ( #7989 ), #18060, .T. ) ;
#2344=ADVANCED_FACE ( 'NONE', ( #13865 ), #677, .F. ) ;
#2346=CARTESIAN_POINT ( 'NONE',  ( 65.51436440461340283, 1.984375000000000000, -12.87863775929475985 ) ) ;
#2353=ORIENTED_EDGE ( 'NONE', *, *, #5626, .T. ) ;
#2357=LINE ( 'NONE', #19271, #10550 ) ;
#2363=VECTOR ( 'NONE', #21213, 1000.000000000000000 ) ;
#2367=ORIENTED_EDGE ( 'NONE', *, *, #17924, .F. ) ;
#2370=DIRECTION ( 'NONE',  ( 0.000000000000000000, 1.000000000000000000, 0.000000000000000000 ) ) ;
#2380=CARTESIAN_POINT ( 'NONE',  ( 1.268730000000000135, 23.41816500000000190, 8.609509071587499562 ) ) ;
#2383=LINE ( 'NONE', #15450, #8838 ) ;
#2386=DIRECTION ( 'NONE',  ( 1.000000000000000000, 0.000000000000000000, 0.000000000000000000 ) ) ;
#2389=LINE ( 'NONE', #6846, #11320 ) ;
#2390=DIRECTION ( 'NONE',  ( 0.5734623443633278805, 0.8192319205190407017, 0.000000000000000000 ) ) ;
#2402=DIRECTION ( 'NONE',  ( 1.000000000000000000, 0.000000000000000000, 0.000000000000000000 ) ) ;
#2412=CARTESIAN_POINT ( 'NONE',  ( -1.848761088705630051, 23.41816500000000190, 7.884515871828260636 ) ) ;
#2415=ORIENTED_EDGE ( 'NONE', *, *, #7631, .T. ) ;
#2429=VERTEX_POINT ( 'NONE', #5772 ) ;
#2434=VERTEX_POINT ( 'NONE', #14082 ) ;
#2465=EDGE_LOOP ( 'NONE', ( #13573, #15352 ) ) ;
#2484=AXIS2_PLACEMENT_3D ( 'NONE', #7530, #14395, #14186 ) ;
#2485=ORIENTED_EDGE ( 'NONE', *, *, #1311, .F. ) ;
#2487=EDGE_CURVE ( 'NONE', #5219, #13475, #12963, .T. ) ;
#2504=DIRECTION ( 'NONE',  ( 0.000000000000000000, 1.000000000000000000, 0.000000000000000000 ) ) ;
#2512=CARTESIAN_POINT ( 'NONE',  ( 31.75000000000000000, 32.54502000000000095, -4.317999999999999616 ) ) ;
#2519=CIRCLE ( 'NONE', #11700, 0.3962400000000010358 ) ;
#2522=CARTESIAN_POINT ( 'NONE',  ( 2.063750000000000195, 30.56064500000000095, -19.71675000000000111 ) ) ;
#2532=CARTESIAN_POINT ( 'NONE',  ( 46.03750000000000142, 30.56064500000000095, -10.31874999999999964 ) ) ;
#2533=DIRECTION ( 'NONE',  ( 0.9579671649362032637, 0.000000000000000000, -0.2868778675745010664 ) ) ;
#2534=CARTESIAN_POINT ( 'NONE',  ( 1.952969610814715207, 23.80837275291289856, 8.731249999999999289 ) ) ;
#2537=VERTEX_POINT ( 'NONE', #11399 ) ;
#2542=ORIENTED_EDGE ( 'NONE', *, *, #1704, .T. ) ;
#2546=CARTESIAN_POINT ( 'NONE',  ( 29.36874999999999858, 9.921875000000000000, 10.71562499999999929 ) ) ;
#2570=CARTESIAN_POINT ( 'NONE',  ( 29.36874999999999858, 9.921875000000000000, 8.731249999999999289 ) ) ;
#2578=CARTESIAN_POINT ( 'NONE',  ( 23.76786555786699751, 0.8616843459004039918, 10.36815399131119975 ) ) ;
#2581=DIRECTION ( 'NONE',  ( 0.000000000000000000, 0.000000000000000000, 1.000000000000000000 ) ) ;
#2584=DIRECTION ( 'NONE',  ( 1.000000000000000000, 0.000000000000000000, 0.000000000000000000 ) ) ;
#2585=AXIS2_PLACEMENT_3D ( 'NONE', #20791, #2680, #21025 ) ;
#2588=CIRCLE ( 'NONE', #8234, 0.3962399999999990929 ) ;
#2591=CARTESIAN_POINT ( 'NONE',  ( 201.9384738932629944, 1.983739999999999837, 8.731885000000000119 ) ) ;
#2604=CARTESIAN_POINT ( 'NONE',  ( 26.59062499999999929, 26.59189500000000095, 8.731249999999999289 ) ) ;
#2609=ORIENTED_EDGE ( 'NONE', *, *, #7352, .F. ) ;
#2611=DIRECTION ( 'NONE',  ( 0.000000000000000000, -1.000000000000000000, 0.000000000000000000 ) ) ;
#2613=ORIENTED_EDGE ( 'NONE', *, *, #11173, .F. ) ;
#2618=FACE_OUTER_BOUND ( 'NONE', #4833, .T. ) ;
#2620=EDGE_CURVE ( 'NONE', #6460, #19683, #14276, .T. ) ;
#2638=ORIENTED_EDGE ( 'NONE', *, *, #10240, .F. ) ;
#2641=AXIS2_PLACEMENT_3D ( 'NONE', #818, #7341, #9202 ) ;
#2643=EDGE_CURVE ( 'NONE', #5275, #11489, #6737, .T. ) ;
#2680=DIRECTION ( 'NONE',  ( -1.000000000000000000, 0.000000000000000000, 0.000000000000000000 ) ) ;
#2688=ORIENTED_EDGE ( 'NONE', *, *, #21779, .F. ) ;
#2692=DIRECTION ( 'NONE',  ( 1.000000000000000000, 0.000000000000000000, 0.000000000000000000 ) ) ;
#2694=EDGE_LOOP ( 'NONE', ( #281, #4609, #228, #6807 ) ) ;
#2699=DIRECTION ( 'NONE',  ( 0.000000000000000000, 1.000000000000000000, 0.000000000000000000 ) ) ;
#2702=DIRECTION ( 'NONE',  ( 0.000000000000000000, 1.000000000000000000, 0.000000000000000000 ) ) ;
#2708=EDGE_LOOP ( 'NONE', ( #17112, #5494, #20962, #13650, #10840, #11675, #14095 ) ) ;
#2714=VERTEX_POINT ( 'NONE', #4866 ) ;
#2716=CARTESIAN_POINT ( 'NONE',  ( 1.954387715434429795, 8.736780638212259475, 10.71562499999999929 ) ) ;
#2722=VERTEX_POINT ( 'NONE', #15278 ) ;
#2736=ORIENTED_EDGE ( 'NONE', *, *, #2262, .T. ) ;
#2739=ORIENTED_EDGE ( 'NONE', *, *, #1751, .T. ) ;
#2743=VERTEX_POINT ( 'NONE', #9947 ) ;
#2747=FACE_OUTER_BOUND ( 'NONE', #9626, .T. ) ;
#2753=LINE ( 'NONE', #18229, #11053 ) ;
#2761=CARTESIAN_POINT ( 'NONE',  ( -12.30312499999999964, 1.984057500000000251, 10.71562499999999929 ) ) ;
#2770=EDGE_CURVE ( 'NONE', #7013, #4043, #15933, .T. ) ;
#2774=CARTESIAN_POINT ( 'NONE',  ( -13.49374999999999858, 0.000000000000000000, 0.000000000000000000 ) ) ;
#2780=PLANE ( 'NONE',  #4942 ) ;
#2789=CARTESIAN_POINT ( 'NONE',  ( 27.48935845518379750, 1.313173473011783887, 10.59903018670800101 ) ) ;
#2790=EDGE_CURVE ( 'NONE', #19275, #2434, #17464, .T. ) ;
#2795=ORIENTED_EDGE ( 'NONE', *, *, #15047, .T. ) ;
#2810=CARTESIAN_POINT ( 'NONE',  ( 46.03750000000000142, 0.000000000000000000, -10.31874999999999964 ) ) ;
#2821=DIRECTION ( 'NONE',  ( 0.9997303917939455165, 0.000000000000000000, 0.02321946863139149123 ) ) ;
#2822=VERTEX_POINT ( 'NONE', #14277 ) ;
#2823=LINE ( 'NONE', #7794, #3572 ) ;
#2825=ORIENTED_EDGE ( 'NONE', *, *, #14435, .T. ) ;
#2829=CIRCLE ( 'NONE', #8461, 22.02656249999999005 ) ;
#2830=ORIENTED_EDGE ( 'NONE', *, *, #18151, .F. ) ;
#2835=CYLINDRICAL_SURFACE ( 'NONE', #11310, 0.3962399999999988154 ) ;
#2838=CARTESIAN_POINT ( 'NONE',  ( 0.02083138522551555155, 20.24316500000000119, 7.210477125664100484 ) ) ;
#2840=ORIENTED_EDGE ( 'NONE', *, *, #10744, .F. ) ;
#2850=CIRCLE ( 'NONE', #15217, 1.984374999999998890 ) ;
#2851=ORIENTED_EDGE ( 'NONE', *, *, #17729, .T. ) ;
#2861=DIRECTION ( 'NONE',  ( 1.000000000000000000, 0.000000000000000000, 0.000000000000000000 ) ) ;
#2866=DIRECTION ( 'NONE',  ( 0.000000000000000000, 1.000000000000000000, 0.000000000000000000 ) ) ;
#2869=CARTESIAN_POINT ( 'NONE',  ( 66.87634738983680904, 32.54502000000000095, 3.497859541731999755 ) ) ;
#2892=EDGE_LOOP ( 'NONE', ( #18348, #7290, #17455, #8127 ) ) ;
#2894=FACE_OUTER_BOUND ( 'NONE', #10046, .T. ) ;
#2897=ORIENTED_EDGE ( 'NONE', *, *, #21417, .T. ) ;
#2905=CIRCLE ( 'NONE', #17744, 9.524999999999998579 ) ;
#2916=DIRECTION ( 'NONE',  ( 0.000000000000000000, 1.000000000000000000, 0.000000000000000000 ) ) ;
#2920=DIRECTION ( 'NONE',  ( 0.000000000000000000, -1.000000000000000000, 0.000000000000000000 ) ) ;
#2922=EDGE_CURVE ( 'NONE', #4819, #13956, #3759, .T. ) ;
#2923=LINE ( 'NONE', #14541, #78 ) ;
#2929=DIRECTION ( 'NONE',  ( 0.000000000000000000, 1.000000000000000000, 0.000000000000000000 ) ) ;
#2931=CARTESIAN_POINT ( 'NONE',  ( 23.41562500000000213, 0.000000000000000000, 5.159374999999999822 ) ) ;
#2932=VERTEX_POINT ( 'NONE', #9151 ) ;
#2934=DIRECTION ( 'NONE',  ( 1.000000000000000000, 0.000000000000000000, 0.000000000000000000 ) ) ;
#2935=CIRCLE ( 'NONE', #817, 3.968750000000000000 ) ;
#2942=DIRECTION ( 'NONE',  ( 0.000000000000000000, 0.000000000000000000, -1.000000000000000000 ) ) ;
#2948=ORIENTED_EDGE ( 'NONE', *, *, #16191, .F. ) ;
#2952=DIRECTION ( 'NONE',  ( -0.9579671649362033747, 0.000000000000000000, 0.2868778675745011775 ) ) ;
#2958=VERTEX_POINT ( 'NONE', #7941 ) ;
#2960=DIRECTION ( 'NONE',  ( 0.000000000000000000, 1.000000000000000000, 0.000000000000000000 ) ) ;
#2965=CYLINDRICAL_SURFACE ( 'NONE', #18054, 1.983740000000001169 ) ;
#2969=ORIENTED_EDGE ( 'NONE', *, *, #8997, .F. ) ;
#2974=EDGE_CURVE ( 'NONE', #4834, #14162, #12939, .T. ) ;
#2988=ORIENTED_EDGE ( 'NONE', *, *, #8997, .T. ) ;
#2996=CYLINDRICAL_SURFACE ( 'NONE', #1774, 0.3962399999999990929 ) ;
#2998=VECTOR ( 'NONE', #2533, 1000.000000000000227 ) ;
#3004=DIRECTION ( 'NONE',  ( -0.2868778675745011220, 0.000000000000000000, -0.9579671649362033747 ) ) ;
#3005=VERTEX_POINT ( 'NONE', #17899 ) ;
#3024=AXIS2_PLACEMENT_3D ( 'NONE', #18003, #11482, #7943 ) ;
#3026=EDGE_CURVE ( 'NONE', #1402, #6719, #19648, .T. ) ;
#3036=ORIENTED_EDGE ( 'NONE', *, *, #14919, .F. ) ;
#3051=ORIENTED_EDGE ( 'NONE', *, *, #843, .F. ) ;
#3065=ORIENTED_EDGE ( 'NONE', *, *, #10197, .T. ) ;
#3074=ADVANCED_FACE ( 'NONE', ( #2747 ), #6388, .F. ) ;
#3077=CARTESIAN_POINT ( 'NONE',  ( 46.03750000000000142, 0.000000000000000000, -10.31874999999999964 ) ) ;
#3083=LINE ( 'NONE', #6390, #13266 ) ;
#3108=CARTESIAN_POINT ( 'NONE',  ( 29.76562500000000000, 30.56064500000000095, -4.317999999999999616 ) ) ;
#3117=VECTOR ( 'NONE', #17381, 1000.000000000000000 ) ;
#3121=DIRECTION ( 'NONE',  ( 0.000000000000000000, 0.000000000000000000, 1.000000000000000000 ) ) ;
#3123=PLANE ( 'NONE',  #7204 ) ;
#3131=DIRECTION ( 'NONE',  ( -1.000000000000000000, 0.000000000000000000, 0.000000000000000000 ) ) ;
#3135=ORIENTED_EDGE ( 'NONE', *, *, #2620, .F. ) ;
#3139=ORIENTED_EDGE ( 'NONE', *, *, #11678, .F. ) ;
#3147=ORIENTED_EDGE ( 'NONE', *, *, #21018, .T. ) ;
#3151=DIRECTION ( 'NONE',  ( -1.000000000000000000, 0.000000000000000000, 0.000000000000000000 ) ) ;
#3154=DIRECTION ( 'NONE',  ( -0.9579671649362032637, 0.000000000000000000, 0.2868778675745010664 ) ) ;
#3163=EDGE_LOOP ( 'NONE', ( #18876, #2795, #11472, #13590 ) ) ;
#3171=VECTOR ( 'NONE', #4795, 1000.000000000000000 ) ;
#3172=ORIENTED_EDGE ( 'NONE', *, *, #5270, .T. ) ;
#3174=ADVANCED_FACE ( 'NONE', ( #15038 ), #16574, .F. ) ;
#3175=VECTOR ( 'NONE', #9870, 1000.000000000000000 ) ;
#3187=VECTOR ( 'NONE', #10703, 1000.000000000000000 ) ;
#3188=EDGE_CURVE ( 'NONE', #6627, #5674, #16681, .T. ) ;
#3190=CARTESIAN_POINT ( 'NONE',  ( -17.46249999999999858, 1.984375000000000000, 0.000000000000000000 ) ) ;
#3195=ORIENTED_EDGE ( 'NONE', *, *, #15367, .T. ) ;
#3199=ORIENTED_EDGE ( 'NONE', *, *, #5708, .T. ) ;
#3201=DIRECTION ( 'NONE',  ( 0.2868778675745010664, 0.000000000000000000, 0.9579671649362032637 ) ) ;
#3212=EDGE_CURVE ( 'NONE', #20891, #12179, #162, .T. ) ;
#3217=DIRECTION ( 'NONE',  ( 0.000000000000000000, -1.000000000000000000, 0.000000000000000000 ) ) ;
#3221=ORIENTED_EDGE ( 'NONE', *, *, #17405, .T. ) ;
#3227=CIRCLE ( 'NONE', #14540, 0.3962400000000008138 ) ;
#3232=VECTOR ( 'NONE', #4382, 1000.000000000000000 ) ;
#3235=CARTESIAN_POINT ( 'NONE',  ( 6.585898268469219552, 32.54502000000000095, 4.694966092919240275 ) ) ;
#3243=AXIS2_PLACEMENT_3D ( 'NONE', #3108, #21783, #16394 ) ;
#3249=CIRCLE ( 'NONE', #17383, 9.524999999999998579 ) ;
#3254=DIRECTION ( 'NONE',  ( 0.000000000000000000, 1.000000000000000000, 0.000000000000000000 ) ) ;
#3258=DIRECTION ( 'NONE',  ( -0.9579671649362032637, 0.000000000000000000, 0.2868778675745010664 ) ) ;
#3268=VERTEX_POINT ( 'NONE', #3706 ) ;
#3270=AXIS2_PLACEMENT_3D ( 'NONE', #6464, #9767, #6780 ) ;
#3272=ORIENTED_EDGE ( 'NONE', *, *, #18097, .T. ) ;
#3284=LINE ( 'NONE', #1502, #22 ) ;
#3287=VECTOR ( 'NONE', #7685, 1000.000000000000114 ) ;
#3289=AXIS2_PLACEMENT_3D ( 'NONE', #1672, #10086, #3454 ) ;
#3292=ORIENTED_EDGE ( 'NONE', *, *, #8367, .T. ) ;
#3294=VERTEX_POINT ( 'NONE', #15441 ) ;
#3297=CIRCLE ( 'NONE', #19863, 3.970019999999998550 ) ;
#3309=DIRECTION ( 'NONE',  ( 0.9999603561554373243, 0.000000000000000000, -0.008904275236710241376 ) ) ;
#3311=CARTESIAN_POINT ( 'NONE',  ( 28.97711086133420366, 30.56064500000000095, -10.31874999999999964 ) ) ;
#3313=AXIS2_PLACEMENT_3D ( 'NONE', #14147, #10473, #7374 ) ;
#3318=VERTEX_POINT ( 'NONE', #11101 ) ;
#3320=CARTESIAN_POINT ( 'NONE',  ( 1.268730000000000135, 23.41816500000000190, 10.65596716962832069 ) ) ;
#3322=ORIENTED_EDGE ( 'NONE', *, *, #12917, .T. ) ;
#3323=ADVANCED_FACE ( 'NONE', ( #14009 ), #5801, .T. ) ;
#3333=VECTOR ( 'NONE', #4968, 1000.000000000000227 ) ;
#3348=( NAMED_UNIT ( * ) SI_UNIT ( $, .STERADIAN. ) SOLID_ANGLE_UNIT ( ) );
#3356=DIRECTION ( 'NONE',  ( 0.000000000000000000, 1.000000000000000000, 0.000000000000000000 ) ) ;
#3366=ORIENTED_EDGE ( 'NONE', *, *, #13040, .F. ) ;
#3382=VECTOR ( 'NONE', #16625, 1000.000000000000227 ) ;
#3384=CARTESIAN_POINT ( 'NONE',  ( 2.063750000000000195, 2.380615000000000148, 8.731249999999999289 ) ) ;
#3394=DIRECTION ( 'NONE',  ( 1.000000000000000000, 0.000000000000000000, 0.000000000000000000 ) ) ;
#3402=DIRECTION ( 'NONE',  ( -1.000000000000000000, 0.000000000000000000, 0.000000000000000000 ) ) ;
#3407=DIRECTION ( 'NONE',  ( -1.000000000000000000, 0.000000000000000000, 0.000000000000000000 ) ) ;
#3408=CARTESIAN_POINT ( 'NONE',  ( 65.67421548912699336, 0.000000000000000000, -10.93409647675949969 ) ) ;
#3418=ORIENTED_EDGE ( 'NONE', *, *, #6294, .T. ) ;
#3419=FACE_OUTER_BOUND ( 'NONE', #2151, .T. ) ;
#3430=AXIS2_PLACEMENT_3D ( 'NONE', #10247, #15695, #13929 ) ;
#3431=VERTEX_POINT ( 'NONE', #9328 ) ;
#3448=VECTOR ( 'NONE', #955, 1000.000000000000000 ) ;
#3454=DIRECTION ( 'NONE',  ( 0.9997303917939455165, 0.000000000000000000, 0.02321946863139149123 ) ) ;
#3459=EDGE_CURVE ( 'NONE', #4834, #6054, #5436, .T. ) ;
#3474=DIRECTION ( 'NONE',  ( 0.000000000000000000, 1.000000000000000000, 0.000000000000000000 ) ) ;
#3492=FACE_OUTER_BOUND ( 'NONE', #771, .T. ) ;
#3510=AXIS2_PLACEMENT_3D ( 'NONE', #19713, #12669, #11000 ) ;
#3513=CARTESIAN_POINT ( 'NONE',  ( 65.51436440461340283, 32.54502000000000095, -12.87863775929475985 ) ) ;
#3518=VERTEX_POINT ( 'NONE', #16738 ) ;
#3523=ORIENTED_EDGE ( 'NONE', *, *, #7734, .F. ) ;
#3527=EDGE_LOOP ( 'NONE', ( #2092, #21268, #2367, #10870 ) ) ;
#3532=CYLINDRICAL_SURFACE ( 'NONE', #5092, 3.970019999999998550 ) ;
#3533=DIRECTION ( 'NONE',  ( 0.000000000000000000, 1.000000000000000000, 0.000000000000000000 ) ) ;
#3548=VECTOR ( 'NONE', #20949, 1000.000000000000000 ) ;
#3549=ORIENTED_EDGE ( 'NONE', *, *, #8954, .F. ) ;
#3553=CARTESIAN_POINT ( 'NONE',  ( -29.36874999999999858, 1.983739999999999837, 10.71562499999999929 ) ) ;
#3554=CARTESIAN_POINT ( 'NONE',  ( 1.952969610814715207, 74.97070807199999365, 6.747510000000000119 ) ) ;
#3555=VECTOR ( 'NONE', #14730, 1000.000000000000000 ) ;
#3563=EDGE_CURVE ( 'NONE', #15983, #1266, #4052, .T. ) ;
#3572=VECTOR ( 'NONE', #2942, 1000.000000000000000 ) ;
#3576=ORIENTED_EDGE ( 'NONE', *, *, #15564, .T. ) ;
#3580=ORIENTED_EDGE ( 'NONE', *, *, #21423, .T. ) ;
#3583=DIRECTION ( 'NONE',  ( 0.000000000000000000, 0.000000000000000000, 1.000000000000000000 ) ) ;
#3586=AXIS2_PLACEMENT_3D ( 'NONE', #2532, #16041, #17571 ) ;
#3589=EDGE_CURVE ( 'NONE', #16780, #8026, #3789, .T. ) ;
#3601=VECTOR ( 'NONE', #17795, 1000.000000000000000 ) ;
#3605=DIRECTION ( 'NONE',  ( 0.000000000000000000, 1.000000000000000000, 0.000000000000000000 ) ) ;
#3606=DIRECTION ( 'NONE',  ( -1.000000000000000000, 0.000000000000000000, 0.000000000000000000 ) ) ;
#3608=CARTESIAN_POINT ( 'NONE',  ( 21.03437500000000071, 32.54502000000000095, 5.159374999999999822 ) ) ;
#3609=EDGE_LOOP ( 'NONE', ( #3549, #3366, #2243, #17336 ) ) ;
#3612=DIRECTION ( 'NONE',  ( 0.9579671649362034858, 0.000000000000000000, -0.2868778675745011220 ) ) ;
#3613=ORIENTED_EDGE ( 'NONE', *, *, #12901, .F. ) ;
#3615=EDGE_CURVE ( 'NONE', #12583, #4819, #18589, .T. ) ;
#3623=VECTOR ( 'NONE', #3606, 1000.000000000000000 ) ;
#3627=CYLINDRICAL_SURFACE ( 'NONE', #12472, 3.968750000000000000 ) ;
#3628=DIRECTION ( 'NONE',  ( 0.000000000000000000, 0.000000000000000000, -1.000000000000000000 ) ) ;
#3629=LINE ( 'NONE', #10476, #3187 ) ;
#3645=CARTESIAN_POINT ( 'NONE',  ( -23.01875000000000071, 32.54502000000000095, -3.968750000000000000 ) ) ;
#3646=VECTOR ( 'NONE', #5382, 1000.000000000000000 ) ;
#3648=LINE ( 'NONE', #1753, #20606 ) ;
#3658=AXIS2_PLACEMENT_3D ( 'NONE', #3077, #9800, #8144 ) ;
#3663=ORIENTED_EDGE ( 'NONE', *, *, #18069, .T. ) ;
#3679=DIRECTION ( 'NONE',  ( 0.000000000000000000, 1.000000000000000000, 0.000000000000000000 ) ) ;
#3695=CARTESIAN_POINT ( 'NONE',  ( 2.063750000000000195, 30.56064500000000095, 8.335010000000000474 ) ) ;
#3700=VECTOR ( 'NONE', #3679, 1000.000000000000000 ) ;
#3706=CARTESIAN_POINT ( 'NONE',  ( 49.81956284419040060, 32.54502000000000095, 11.98436472153758103 ) ) ;
#3711=ADVANCED_FACE ( 'NONE', ( #13391 ), #21881, .F. ) ;
#3723=CARTESIAN_POINT ( 'NONE',  ( -157.1365884395040098, 9.924415000000001541, 46.81779025872040023 ) ) ;
#3724=EDGE_LOOP ( 'NONE', ( #10788, #16458, #5932, #4732, #974, #10027 ) ) ;
#3732=DIRECTION ( 'NONE',  ( 0.9999999998269335499, -1.860465115920061245E-05, 0.000000000000000000 ) ) ;
#3738=FACE_OUTER_BOUND ( 'NONE', #18756, .T. ) ;
#3742=CARTESIAN_POINT ( 'NONE',  ( -2.028188046367890074, 9.129395000000000593, 0.3682158094503220069 ) ) ;
#3751=ORIENTED_EDGE ( 'NONE', *, *, #18097, .F. ) ;
#3759=LINE ( 'NONE', #17572, #21311 ) ;
#3761=FACE_OUTER_BOUND ( 'NONE', #9032, .T. ) ;
#3771=EDGE_CURVE ( 'NONE', #1261, #12179, #18194, .T. ) ;
#3776=ORIENTED_EDGE ( 'NONE', *, *, #7706, .T. ) ;
#3777=LINE ( 'NONE', #13852, #14159 ) ;
#3789=LINE ( 'NONE', #18698, #17107 ) ;
#3813=VECTOR ( 'NONE', #4286, 1000.000000000000000 ) ;
#3816=CARTESIAN_POINT ( 'NONE',  ( 31.75000000000000000, 32.54502000000000095, -4.317999999999999616 ) ) ;
#3819=ADVANCED_FACE ( 'NONE', ( #20213 ), #104, .F. ) ;
#3829=EDGE_LOOP ( 'NONE', ( #4200, #14448, #19212, #13377, #10019 ) ) ;
#3835=CARTESIAN_POINT ( 'NONE',  ( -4.157227781567939928, 9.924415000000001541, 0.1758860224507720060 ) ) ;
#3839=ADVANCED_FACE ( 'NONE', ( #3761 ), #1547, .T. ) ;
#3843=CARTESIAN_POINT ( 'NONE',  ( 1.883505690267595956, 8.857556300445232011, 10.71562500000000107 ) ) ;
#3859=AXIS2_PLACEMENT_3D ( 'NONE', #16184, #17331, #8801 ) ;
#3861=ORIENTED_EDGE ( 'NONE', *, *, #15671, .F. ) ;
#3875=VERTEX_POINT ( 'NONE', #18995 ) ;
#3881=VERTEX_POINT ( 'NONE', #7293 ) ;
#3883=DIRECTION ( 'NONE',  ( 0.000000000000000000, 1.000000000000000000, 0.000000000000000000 ) ) ;
#3885=ORIENTED_EDGE ( 'NONE', *, *, #14904, .T. ) ;
#3903=CARTESIAN_POINT ( 'NONE',  ( 66.03921914090641110, -42.42568807200000691, -11.33033647675950029 ) ) ;
#3914=ORIENTED_EDGE ( 'NONE', *, *, #2240, .T. ) ;
#3915=LINE ( 'NONE', #3695, #14894 ) ;
#3924=CYLINDRICAL_SURFACE ( 'NONE', #6838, 0.3962400000000008138 ) ;
#3927=VECTOR ( 'NONE', #9899, 1000.000000000000000 ) ;
#3930=PLANE ( 'NONE',  #12010 ) ;
#3937=CARTESIAN_POINT ( 'NONE',  ( 36.51250000000000284, 0.000000000000000000, -10.31875000000000142 ) ) ;
#3944=VERTEX_POINT ( 'NONE', #19222 ) ;
#3959=ORIENTED_EDGE ( 'NONE', *, *, #12542, .T. ) ;
#3961=CIRCLE ( 'NONE', #16331, 6.349999999999999645 ) ;
#3992=CARTESIAN_POINT ( 'NONE',  ( 29.37324403177899868, 30.56064500000000095, -10.70578951775076071 ) ) ;
#3994=ORIENTED_EDGE ( 'NONE', *, *, #4822, .F. ) ;
#3997=DIRECTION ( 'NONE',  ( 0.000000000000000000, -1.000000000000000000, 0.000000000000000000 ) ) ;
#4010=VECTOR ( 'NONE', #8521, 1000.000000000000000 ) ;
#4018=EDGE_LOOP ( 'NONE', ( #3147, #1747 ) ) ;
#4020=AXIS2_PLACEMENT_3D ( 'NONE', #11023, #13136, #9684 ) ;
#4022=EDGE_CURVE ( 'NONE', #5923, #6054, #5451, .T. ) ;
#4043=VERTEX_POINT ( 'NONE', #13953 ) ;
#4052=CIRCLE ( 'NONE', #16417, 0.7950199999999997269 ) ;
#4066=ORIENTED_EDGE ( 'NONE', *, *, #2487, .T. ) ;
#4069=DIRECTION ( 'NONE',  ( 0.000000000000000000, -1.000000000000000000, 0.000000000000000000 ) ) ;
#4077=VERTEX_POINT ( 'NONE', #17901 ) ;
#4082=DIRECTION ( 'NONE',  ( 0.000000000000000000, 0.000000000000000000, 1.000000000000000000 ) ) ;
#4091=AXIS2_PLACEMENT_3D ( 'NONE', #12998, #3131, #6561 ) ;
#4095=EDGE_CURVE ( 'NONE', #19126, #9142, #6879, .T. ) ;
#4097=EDGE_CURVE ( 'NONE', #13820, #966, #9700, .T. ) ;
#4103=DIRECTION ( 'NONE',  ( 0.5734623443633278805, 0.8192319205190407017, 0.000000000000000000 ) ) ;
#4114=FACE_OUTER_BOUND ( 'NONE', #4512, .T. ) ;
#4117=DIRECTION ( 'NONE',  ( 0.000000000000000000, 0.000000000000000000, -1.000000000000000000 ) ) ;
#4119=ORIENTED_EDGE ( 'NONE', *, *, #8322, .F. ) ;
#4120=CARTESIAN_POINT ( 'NONE',  ( 66.03921914090641110, 1.984375000000000000, -10.93409647675949969 ) ) ;
#4129=EDGE_CURVE ( 'NONE', #21761, #21868, #3083, .T. ) ;
#4132=FACE_BOUND ( 'NONE', #11763, .T. ) ;
#4138=CYLINDRICAL_SURFACE ( 'NONE', #9858, 1.983739999999999837 ) ;
#4147=ORIENTED_EDGE ( 'NONE', *, *, #11526, .T. ) ;
#4168=FACE_OUTER_BOUND ( 'NONE', #16376, .T. ) ;
#4170=CARTESIAN_POINT ( 'NONE',  ( 49.09065990372640442, 0.000000000000000000, -26.70549589918839928 ) ) ;
#4180=VERTEX_POINT ( 'NONE', #1302 ) ;
#4184=ORIENTED_EDGE ( 'NONE', *, *, #18151, .T. ) ;
#4190=CARTESIAN_POINT ( 'NONE',  ( 1.535814226138735528, 23.46100396823117862, 8.688060833667504923 ) ) ;
#4198=VECTOR ( 'NONE', #7115, 1000.000000000000000 ) ;
#4200=ORIENTED_EDGE ( 'NONE', *, *, #14543, .F. ) ;
#4207=ORIENTED_EDGE ( 'NONE', *, *, #10301, .T. ) ;
#4216=AXIS2_PLACEMENT_3D ( 'NONE', #14320, #20804, #1019 ) ;
#4227=CARTESIAN_POINT ( 'NONE',  ( 65.64431122251959039, 32.54502000000000095, -11.29787305743958115 ) ) ;
#4233=ORIENTED_EDGE ( 'NONE', *, *, #17908, .F. ) ;
#4235=CARTESIAN_POINT ( 'NONE',  ( 25.99163424860619642, 1.095943520706746055, 10.50611347932359863 ) ) ;
#4239=EDGE_CURVE ( 'NONE', #1356, #11142, #17495, .T. ) ;
#4240=CARTESIAN_POINT ( 'NONE',  ( -1.345424459097947834, 20.24316500000000119, 2.648158502653860324 ) ) ;
#4241=AXIS2_PLACEMENT_3D ( 'NONE', #5333, #20143, #18604 ) ;
#4243=DIRECTION ( 'NONE',  ( 1.000000000000000000, 0.000000000000000000, 0.000000000000000000 ) ) ;
#4245=ORIENTED_EDGE ( 'NONE', *, *, #8143, .F. ) ;
#4247=ADVANCED_FACE ( 'NONE', ( #13048 ), #74, .F. ) ;
#4251=DIRECTION ( 'NONE',  ( 0.000000000000000000, 0.000000000000000000, -1.000000000000000000 ) ) ;
#4256=CIRCLE ( 'NONE', #21541, 9.524999999999998579 ) ;
#4257=EDGE_LOOP ( 'NONE', ( #1025, #7550 ) ) ;
#4274=DIRECTION ( 'NONE',  ( 0.000000000000000000, 1.000000000000000000, 0.000000000000000000 ) ) ;
#4276=CIRCLE ( 'NONE', #5670, 1.983739999999999837 ) ;
#4282=ORIENTED_EDGE ( 'NONE', *, *, #4842, .F. ) ;
#4286=DIRECTION ( 'NONE',  ( 0.000000000000000000, -1.000000000000000000, 0.000000000000000000 ) ) ;
#4290=VECTOR ( 'NONE', #2611, 1000.000000000000000 ) ;
#4299=ORIENTED_EDGE ( 'NONE', *, *, #12848, .F. ) ;
#4307=CARTESIAN_POINT ( 'NONE',  ( 28.97711086133420366, 30.56064500000000095, -10.71499000000000024 ) ) ;
#4312=CARTESIAN_POINT ( 'NONE',  ( 29.76562500000000000, 32.54502000000000095, -4.317999999999999616 ) ) ;
#4314=DIRECTION ( 'NONE',  ( -1.000000000000000000, 0.000000000000000000, 0.000000000000000000 ) ) ;
#4316=ORIENTED_EDGE ( 'NONE', *, *, #5859, .T. ) ;
#4318=CARTESIAN_POINT ( 'NONE',  ( 28.97711086133420366, 30.56064500000000095, -10.31874999999999964 ) ) ;
#4321=ORIENTED_EDGE ( 'NONE', *, *, #3212, .T. ) ;
#4322=ORIENTED_EDGE ( 'NONE', *, *, #15590, .F. ) ;
#4325=AXIS2_PLACEMENT_3D ( 'NONE', #1629, #21864, #15256 ) ;
#4331=LINE ( 'NONE', #7641, #14625 ) ;
#4343=ORIENTED_EDGE ( 'NONE', *, *, #5346, .F. ) ;
#4346=CIRCLE ( 'NONE', #15297, 9.524999999999998579 ) ;
#4349=CARTESIAN_POINT ( 'NONE',  ( 20.47138736203545051, 0.6100621568841679832, 10.16364511138895921 ) ) ;
#4350=ADVANCED_FACE ( 'NONE', ( #13693 ), #20393, .F. ) ;
#4361=CARTESIAN_POINT ( 'NONE',  ( 29.36874999999999858, 9.921875000000000000, 8.731249999999999289 ) ) ;
#4368=ORIENTED_EDGE ( 'NONE', *, *, #21688, .T. ) ;
#4375=LINE ( 'NONE', #6015, #5260 ) ;
#4382=DIRECTION ( 'NONE',  ( 0.000000000000000000, -1.000000000000000000, 0.000000000000000000 ) ) ;
#4384=DIRECTION ( 'NONE',  ( 1.000000000000000000, 0.000000000000000000, 0.000000000000000000 ) ) ;
#4386=EDGE_LOOP ( 'NONE', ( #19555, #18791, #19167, #15736 ) ) ;
#4394=CIRCLE ( 'NONE', #9320, 25.00312500000000426 ) ;
#4395=ADVANCED_FACE ( 'NONE', ( #9916 ), #13370, .F. ) ;
#4400=CYLINDRICAL_SURFACE ( 'NONE', #11987, 16.66875000000000284 ) ;
#4424=VERTEX_POINT ( 'NONE', #20625 ) ;
#4427=LINE ( 'NONE', #11261, #11021 ) ;
#4428=DIRECTION ( 'NONE',  ( 0.000000000000000000, 0.000000000000000000, -1.000000000000000000 ) ) ;
#4429=EDGE_LOOP ( 'NONE', ( #11195, #7844, #18649, #2353 ) ) ;
#4459=CARTESIAN_POINT ( 'NONE',  ( 29.29500096977420043, 1.844679962977120002, 10.71104922697731965 ) ) ;
#4461=DIRECTION ( 'NONE',  ( 0.000000000000000000, -1.000000000000000000, 0.000000000000000000 ) ) ;
#4486=DIRECTION ( 'NONE',  ( 0.000000000000000000, 0.000000000000000000, 1.000000000000000000 ) ) ;
#4488=ORIENTED_EDGE ( 'NONE', *, *, #11302, .F. ) ;
#4490=ORIENTED_EDGE ( 'NONE', *, *, #4798, .T. ) ;
#4496=EDGE_CURVE ( 'NONE', #20164, #1402, #7595, .T. ) ;
#4508=ORIENTED_EDGE ( 'NONE', *, *, #9373, .T. ) ;
#4509=VECTOR ( 'NONE', #17664, 1000.000000000000000 ) ;
#4510=VERTEX_POINT ( 'NONE', #2053 ) ;
#4512=EDGE_LOOP ( 'NONE', ( #11655, #15104, #9971, #11088, #3272 ) ) ;
#4514=ADVANCED_FACE ( 'NONE', ( #1031 ), #14434, .F. ) ;
#4524=CARTESIAN_POINT ( 'NONE',  ( -17.46249999999999858, 16.27314499999999953, 8.731249999999999289 ) ) ;
#4529=DIRECTION ( 'NONE',  ( 0.000000000000000000, 1.000000000000000000, 0.000000000000000000 ) ) ;
#4532=ORIENTED_EDGE ( 'NONE', *, *, #18650, .F. ) ;
#4547=ORIENTED_EDGE ( 'NONE', *, *, #15539, .T. ) ;
#4553=DIRECTION ( 'NONE',  ( -1.000000000000000000, 0.000000000000000000, 0.000000000000000000 ) ) ;
#4559=CARTESIAN_POINT ( 'NONE',  ( 28.90809283614979819, 1.647247860330810054, 10.68704647368243954 ) ) ;
#4581=EDGE_LOOP ( 'NONE', ( #13433, #8731, #3861, #20771, #21272, #14746 ) ) ;
#4591=DIRECTION ( 'NONE',  ( 1.000000000000000000, 0.000000000000000000, 0.000000000000000000 ) ) ;
#4594=AXIS2_PLACEMENT_3D ( 'NONE', #1589, #9765, #21814 ) ;
#4596=CIRCLE ( 'NONE', #10586, 6.349999999999999645 ) ;
#4604=DIRECTION ( 'NONE',  ( 1.000000000000000000, 0.000000000000000000, 0.000000000000000000 ) ) ;
#4605=ORIENTED_EDGE ( 'NONE', *, *, #1413, .T. ) ;
#4608=CARTESIAN_POINT ( 'NONE',  ( 1.268730000000000135, 8.334374999999999645, 10.71562499999999929 ) ) ;
#4609=ORIENTED_EDGE ( 'NONE', *, *, #14486, .T. ) ;
#4613=LINE ( 'NONE', #19965, #10633 ) ;
#4618=AXIS2_PLACEMENT_3D ( 'NONE', #18657, #20409, #20528 ) ;
#4619=ORIENTED_EDGE ( 'NONE', *, *, #665, .T. ) ;
#4630=EDGE_LOOP ( 'NONE', ( #7609, #5405, #11712, #17181, #14479, #11548 ) ) ;
#4631=AXIS2_PLACEMENT_3D ( 'NONE', #10815, #20980, #17889 ) ;
#4634=DIRECTION ( 'NONE',  ( -1.000000000000000000, 0.000000000000000000, 0.000000000000000000 ) ) ;
#4644=ORIENTED_EDGE ( 'NONE', *, *, #7507, .F. ) ;
#4667=ORIENTED_EDGE ( 'NONE', *, *, #1561, .T. ) ;
#4669=CIRCLE ( 'NONE', #15987, 0.3962400000000010358 ) ;
#4677=DIRECTION ( 'NONE',  ( 0.000000000000000000, -1.000000000000000000, 0.000000000000000000 ) ) ;
#4680=SURFACE_STYLE_USAGE ( .BOTH. , #19804 ) ;
#4691=FACE_OUTER_BOUND ( 'NONE', #17436, .T. ) ;
#4694=EDGE_CURVE ( 'NONE', #16263, #18972, #554, .T. ) ;
#4699=DIRECTION ( 'NONE',  ( 0.000000000000000000, 0.000000000000000000, -1.000000000000000000 ) ) ;
#4704=FACE_OUTER_BOUND ( 'NONE', #14698, .T. ) ;
#4718=CIRCLE ( 'NONE', #15317, 2.381250000000001421 ) ;
#4721=EDGE_CURVE ( 'NONE', #4510, #7810, #9856, .T. ) ;
#4722=PLANE ( 'NONE',  #18717 ) ;
#4731=DIRECTION ( 'NONE',  ( 0.000000000000000000, 0.000000000000000000, -1.000000000000000000 ) ) ;
#4732=ORIENTED_EDGE ( 'NONE', *, *, #10056, .T. ) ;
#4736=VERTEX_POINT ( 'NONE', #6658 ) ;
#4740=VECTOR ( 'NONE', #21065, 1000.000000000000000 ) ;
#4742=AXIS2_PLACEMENT_3D ( 'NONE', #21048, #12557, #9433 ) ;
#4748=ORIENTED_EDGE ( 'NONE', *, *, #4909, .T. ) ;
#4750=DIRECTION ( 'NONE',  ( 0.000000000000000000, 1.000000000000000000, 0.000000000000000000 ) ) ;
#4751=DIRECTION ( 'NONE',  ( 0.000000000000000000, 1.000000000000000000, 0.000000000000000000 ) ) ;
#4752=CARTESIAN_POINT ( 'NONE',  ( 54.51779242482700027, 1.984375000000000000, -30.64740209392260084 ) ) ;
#4760=DIRECTION ( 'NONE',  ( 0.000000000000000000, 0.000000000000000000, -1.000000000000000000 ) ) ;
#4764=ADVANCED_FACE ( 'NONE', ( #4691 ), #16519, .F. ) ;
#4769=EDGE_CURVE ( 'NONE', #138, #14162, #18556, .T. ) ;
#4770=FACE_OUTER_BOUND ( 'NONE', #19525, .T. ) ;
#4781=DIRECTION ( 'NONE',  ( 0.000000000000000000, 1.000000000000000000, 0.000000000000000000 ) ) ;
#4785=DIRECTION ( 'NONE',  ( 0.000000000000000000, 0.000000000000000000, 1.000000000000000000 ) ) ;
#4795=DIRECTION ( 'NONE',  ( 0.000000000000000000, 1.000000000000000000, 0.000000000000000000 ) ) ;
#4798=EDGE_CURVE ( 'NONE', #2743, #7667, #6226, .T. ) ;
#4817=DIRECTION ( 'NONE',  ( 1.000000000000000000, 0.000000000000000000, 0.000000000000000000 ) ) ;
#4819=VERTEX_POINT ( 'NONE', #21804 ) ;
#4822=EDGE_CURVE ( 'NONE', #8026, #17335, #6768, .T. ) ;
#4825=LINE ( 'NONE', #9678, #5680 ) ;
#4832=DIRECTION ( 'NONE',  ( 0.000000000000000000, 1.000000000000000000, 0.000000000000000000 ) ) ;
#4833=EDGE_LOOP ( 'NONE', ( #209, #21241, #14980, #16450 ) ) ;
#4834=VERTEX_POINT ( 'NONE', #5434 ) ;
#4835=LINE ( 'NONE', #11570, #1734 ) ;
#4842=EDGE_CURVE ( 'NONE', #6814, #20045, #17165, .T. ) ;
#4843=CARTESIAN_POINT ( 'NONE',  ( 70.64340948846358970, 74.97070807199999365, -10.53785647675949910 ) ) ;
#4844=ORIENTED_EDGE ( 'NONE', *, *, #15319, .F. ) ;
#4846=DIRECTION ( 'NONE',  ( 0.000000000000000000, 0.000000000000000000, -1.000000000000000000 ) ) ;
#4848=DIRECTION ( 'NONE',  ( 0.000000000000000000, -1.000000000000000000, 0.000000000000000000 ) ) ;
#4850=ORIENTED_EDGE ( 'NONE', *, *, #20867, .F. ) ;
#4853=CARTESIAN_POINT ( 'NONE',  ( -13.49374999999999858, 32.54502000000000095, 0.000000000000000000 ) ) ;
#4855=ORIENTED_EDGE ( 'NONE', *, *, #20717, .F. ) ;
#4856=ORIENTED_EDGE ( 'NONE', *, *, #16907, .T. ) ;
#4858=VECTOR ( 'NONE', #894, 1000.000000000000227 ) ;
#4859=DIRECTION ( 'NONE',  ( 0.000000000000000000, 1.000000000000000000, 0.000000000000000000 ) ) ;
#4862=CARTESIAN_POINT ( 'NONE',  ( -2.028188046367890074, 23.41816500000000190, 0.3682158094503220069 ) ) ;
#4866=CARTESIAN_POINT ( 'NONE',  ( 1.952969610814715207, 8.739187247087119914, 8.731249999999999289 ) ) ;
#4881=CYLINDRICAL_SURFACE ( 'NONE', #7395, 0.3962399999999999811 ) ;
#4885=ADVANCED_FACE ( 'NONE', ( #20686 ), #12199, .F. ) ;
#4886=DIRECTION ( 'NONE',  ( 0.2868778675745010664, 0.000000000000000000, 0.9579671649362032637 ) ) ;
#4891=DIRECTION ( 'NONE',  ( 0.000000000000000000, 1.000000000000000000, 0.000000000000000000 ) ) ;
#4893=DIRECTION ( 'NONE',  ( -0.9579671649362034858, -3.931712979385797282E-31, 0.2868778675745011220 ) ) ;
#4901=DIRECTION ( 'NONE',  ( -0.9579671649362032637, 0.000000000000000000, 0.2868778675745010664 ) ) ;
#4908=FACE_OUTER_BOUND ( 'NONE', #5525, .T. ) ;
#4909=EDGE_CURVE ( 'NONE', #7279, #21761, #16464, .T. ) ;
#4916=ORIENTED_EDGE ( 'NONE', *, *, #8047, .T. ) ;
#4927=CARTESIAN_POINT ( 'NONE',  ( 0.05128277951103899640, 30.56064500000000095, 8.896810487299289250 ) ) ;
#4933=VERTEX_POINT ( 'NONE', #10309 ) ;
#4936=ORIENTED_EDGE ( 'NONE', *, *, #8493, .F. ) ;
#4942=AXIS2_PLACEMENT_3D ( 'NONE', #6201, #18155, #16393 ) ;
#4944=DIRECTION ( 'NONE',  ( -1.000000000000000000, 0.000000000000000000, 0.000000000000000000 ) ) ;
#4946=ORIENTED_EDGE ( 'NONE', *, *, #11522, .T. ) ;
#4949=CARTESIAN_POINT ( 'NONE',  ( 0.000000000000000000, 0.000000000000000000, 0.000000000000000000 ) ) ;
#4950=ADVANCED_FACE ( 'NONE', ( #5543 ), #12301, .F. ) ;
#4956=AXIS2_PLACEMENT_3D ( 'NONE', #13094, #9745, #11306 ) ;
#4960=CARTESIAN_POINT ( 'NONE',  ( 54.51779242482700027, 0.000000000000000000, -30.64740209392260084 ) ) ;
#4968=DIRECTION ( 'NONE',  ( 0.9579671649362032637, 0.000000000000000000, -0.2868778675745010664 ) ) ;
#4979=ORIENTED_EDGE ( 'NONE', *, *, #6553, .T. ) ;
#4984=ORIENTED_EDGE ( 'NONE', *, *, #10953, .F. ) ;
#4985=VECTOR ( 'NONE', #14323, 1000.000000000000000 ) ;
#4986=AXIS2_PLACEMENT_3D ( 'NONE', #1389, #2960, #6487 ) ;
#4988=CARTESIAN_POINT ( 'NONE',  ( 1.268730000000000135, 8.334374999999999645, 8.731249999999999289 ) ) ;
#4992=FACE_BOUND ( 'NONE', #11822, .T. ) ;
#5001=DIRECTION ( 'NONE',  ( 1.000000000000000000, 0.000000000000000000, 0.000000000000000000 ) ) ;
#5008=AXIS2_PLACEMENT_3D ( 'NONE', #1737, #19874, #21863 ) ;
#5034=EDGE_CURVE ( 'NONE', #21568, #12037, #19362, .T. ) ;
#5035=ORIENTED_EDGE ( 'NONE', *, *, #10215, .T. ) ;
#5047=CARTESIAN_POINT ( 'NONE',  ( 70.64340948846358970, 30.56064500000000095, -10.53785647675949910 ) ) ;
#5056=VECTOR ( 'NONE', #20233, 1000.000000000000000 ) ;
#5063=ADVANCED_FACE ( 'NONE', ( #7756, #10966, #17837, #21238, #11184 ), #20916, .F. ) ;
#5064=CARTESIAN_POINT ( 'NONE',  ( 50.99913033092320092, 1.984375000000000000, -7.029081061492260751 ) ) ;
#5066=FACE_BOUND ( 'NONE', #12798, .T. ) ;
#5067=CARTESIAN_POINT ( 'NONE',  ( -12.30312499999999964, 2.380615000000000148, 8.731249999999999289 ) ) ;
#5068=CARTESIAN_POINT ( 'NONE',  ( 46.03750000000000142, 0.000000000000000000, -10.31874999999999964 ) ) ;
#5072=ORIENTED_EDGE ( 'NONE', *, *, #3771, .T. ) ;
#5074=FACE_OUTER_BOUND ( 'NONE', #9933, .T. ) ;
#5078=DIRECTION ( 'NONE',  ( 0.000000000000000000, 1.000000000000000000, 0.000000000000000000 ) ) ;
#5082=EDGE_CURVE ( 'NONE', #19124, #19591, #12749, .T. ) ;
#5085=ADVANCED_FACE ( 'NONE', ( #582, #17719 ), #5978, .T. ) ;
#5090=ORIENTED_EDGE ( 'NONE', *, *, #14516, .F. ) ;
#5092=AXIS2_PLACEMENT_3D ( 'NONE', #322, #17241, #20995 ) ;
#5093=DIRECTION ( 'NONE',  ( 0.000000000000000000, 1.000000000000000000, 0.000000000000000000 ) ) ;
#5107=EDGE_CURVE ( 'NONE', #12461, #13767, #15967, .T. ) ;
#5121=CARTESIAN_POINT ( 'NONE',  ( -2.256261688646920227, 9.924415000000001541, -0.3933872460174320240 ) ) ;
#5130=ADVANCED_FACE ( 'NONE', ( #7326 ), #5778, .F. ) ;
#5139=ORIENTED_EDGE ( 'NONE', *, *, #691, .T. ) ;
#5144=CARTESIAN_POINT ( 'NONE',  ( -17.46249999999999858, 0.000000000000000000, 0.000000000000000000 ) ) ;
#5147=DIRECTION ( 'NONE',  ( 0.000000000000000000, -1.000000000000000000, 0.000000000000000000 ) ) ;
#5151=ORIENTED_EDGE ( 'NONE', *, *, #12542, .F. ) ;
#5165=CARTESIAN_POINT ( 'NONE',  ( 65.51436440461340283, 30.56064500000000095, -12.87863775929475985 ) ) ;
#5169=ORIENTED_EDGE ( 'NONE', *, *, #14023, .T. ) ;
#5177=VECTOR ( 'NONE', #1683, 1000.000000000000000 ) ;
#5199=EDGE_CURVE ( 'NONE', #6719, #9795, #1825, .T. ) ;
#5205=AXIS2_PLACEMENT_3D ( 'NONE', #11403, #9731, #11285 ) ;
#5219=VERTEX_POINT ( 'NONE', #20003 ) ;
#5253=LINE ( 'NONE', #20618, #6130 ) ;
#5254=EDGE_LOOP ( 'NONE', ( #1062, #18163, #20420, #19240 ) ) ;
#5257=CARTESIAN_POINT ( 'NONE',  ( 0.02083138522552824973, 12.30439499999999953, 7.210477125664100484 ) ) ;
#5259=CARTESIAN_POINT ( 'NONE',  ( 55.56250000000000000, 0.000000000000000000, -10.31874999999999964 ) ) ;
#5260=VECTOR ( 'NONE', #19510, 1000.000000000000000 ) ;
#5261=EDGE_LOOP ( 'NONE', ( #21498, #11220, #12755, #15152 ) ) ;
#5268=ORIENTED_EDGE ( 'NONE', *, *, #311, .T. ) ;
#5270=EDGE_CURVE ( 'NONE', #11600, #18667, #13140, .T. ) ;
#5275=VERTEX_POINT ( 'NONE', #14850 ) ;
#5276=DIRECTION ( 'NONE',  ( 0.000000000000000000, 1.000000000000000000, 0.000000000000000000 ) ) ;
#5283=CARTESIAN_POINT ( 'NONE',  ( -21.43124999999999858, 0.000000000000000000, -4.860316984116058095E-16 ) ) ;
#5284=DIRECTION ( 'NONE',  ( 0.000000000000000000, 0.000000000000000000, 1.000000000000000000 ) ) ;
#5287=VECTOR ( 'NONE', #3121, 1000.000000000000000 ) ;
#5293=ORIENTED_EDGE ( 'NONE', *, *, #15972, .T. ) ;
#5298=VECTOR ( 'NONE', #8744, 1000.000000000000000 ) ;
#5302=EDGE_LOOP ( 'NONE', ( #11580, #11027, #10818, #12451 ) ) ;
#5306=CYLINDRICAL_SURFACE ( 'NONE', #20750, 16.66875000000000284 ) ;
#5309=VECTOR ( 'NONE', #20207, 1000.000000000000000 ) ;
#5315=AXIS2_PLACEMENT_3D ( 'NONE', #9081, #10646, #14091 ) ;
#5327=EDGE_CURVE ( 'NONE', #2537, #16536, #10287, .T. ) ;
#5328=AXIS2_PLACEMENT_3D ( 'NONE', #19831, #19716, #2821 ) ;
#5333=CARTESIAN_POINT ( 'NONE',  ( 21.43124999999999858, 16.27314499999999953, 8.731249999999999289 ) ) ;
#5340=AXIS2_PLACEMENT_3D ( 'NONE', #8329, #14996, #1684 ) ;
#5346=EDGE_CURVE ( 'NONE', #21849, #16032, #9954, .T. ) ;
#5351=AXIS2_PLACEMENT_3D ( 'NONE', #11406, #7649, #6094 ) ;
#5369=DIRECTION ( 'NONE',  ( 0.000000000000000000, -1.000000000000000000, 0.000000000000000000 ) ) ;
#5370=ORIENTED_EDGE ( 'NONE', *, *, #8955, .F. ) ;
#5371=CARTESIAN_POINT ( 'NONE',  ( -23.01875000000000071, 0.000000000000000000, -10.31874999999999964 ) ) ;
#5374=EDGE_CURVE ( 'NONE', #9016, #13089, #12057, .T. ) ;
#5381=ORIENTED_EDGE ( 'NONE', *, *, #3212, .F. ) ;
#5382=DIRECTION ( 'NONE',  ( 0.000000000000000000, 0.000000000000000000, 1.000000000000000000 ) ) ;
#5401=FACE_OUTER_BOUND ( 'NONE', #8581, .T. ) ;
#5405=ORIENTED_EDGE ( 'NONE', *, *, #10056, .F. ) ;
#5423=DIRECTION ( 'NONE',  ( -0.8193181045417649022, -0.5733392046337750791, 0.000000000000000000 ) ) ;
#5434=CARTESIAN_POINT ( 'NONE',  ( 49.09065990372640442, 30.56064500000000095, -26.70549589918839928 ) ) ;
#5436=CIRCLE ( 'NONE', #12536, 16.66874999999998508 ) ;
#5444=VECTOR ( 'NONE', #6440, 1000.000000000000000 ) ;
#5445=ORIENTED_EDGE ( 'NONE', *, *, #12917, .F. ) ;
#5449=CARTESIAN_POINT ( 'NONE',  ( 26.59062499999999929, 1.984375000000000000, -2.268784209304649746 ) ) ;
#5451=CIRCLE ( 'NONE', #17839, 0.3962400000000008138 ) ;
#5461=CARTESIAN_POINT ( 'NONE',  ( -13.49374999999999858, 1.984375000000000000, 0.000000000000000000 ) ) ;
#5471=EDGE_LOOP ( 'NONE', ( #14394, #14567 ) ) ;
#5477=DIRECTION ( 'NONE',  ( 0.000000000000000000, 1.000000000000000000, -1.313388458492437221E-14 ) ) ;
#5480=EDGE_LOOP ( 'NONE', ( #16344, #516, #19004, #13353 ) ) ;
#5484=LINE ( 'NONE', #14031, #7503 ) ;
#5491=CARTESIAN_POINT ( 'NONE',  ( -17.46249999999999858, 0.000000000000000000, 0.000000000000000000 ) ) ;
#5494=ORIENTED_EDGE ( 'NONE', *, *, #8493, .T. ) ;
#5501=EDGE_LOOP ( 'NONE', ( #12356, #8368, #21108, #2840 ) ) ;
#5519=ORIENTED_EDGE ( 'NONE', *, *, #3459, .F. ) ;
#5520=ORIENTED_EDGE ( 'NONE', *, *, #21503, .F. ) ;
#5525=EDGE_LOOP ( 'NONE', ( #1871, #15386, #17941, #3065 ) ) ;
#5526=ORIENTED_EDGE ( 'NONE', *, *, #8979, .T. ) ;
#5542=DIRECTION ( 'NONE',  ( 1.000000000000000000, 0.000000000000000000, 0.000000000000000000 ) ) ;
#5543=FACE_OUTER_BOUND ( 'NONE', #9438, .T. ) ;
#5548=ORIENTED_EDGE ( 'NONE', *, *, #10174, .F. ) ;
#5552=VECTOR ( 'NONE', #20853, 1000.000000000000000 ) ;
#5558=CARTESIAN_POINT ( 'NONE',  ( -29.36874999999999858, 30.56064500000000095, 8.335010000000000474 ) ) ;
#5563=FACE_OUTER_BOUND ( 'NONE', #120, .T. ) ;
#5585=EDGE_LOOP ( 'NONE', ( #12224, #2485, #18899, #3580 ) ) ;
#5601=CARTESIAN_POINT ( 'NONE',  ( -12.30312499999999964, 1.984375000000000000, 8.335010000000000474 ) ) ;
#5603=CARTESIAN_POINT ( 'NONE',  ( -12.30312499999999964, 1.984375000000000000, 8.335010000000000474 ) ) ;
#5609=VERTEX_POINT ( 'NONE', #14382 ) ;
#5614=ORIENTED_EDGE ( 'NONE', *, *, #4909, .F. ) ;
#5619=AXIS2_PLACEMENT_3D ( 'NONE', #16345, #7602, #7812 ) ;
#5622=CIRCLE ( 'NONE', #10572, 19.05000000000000071 ) ;
#5626=EDGE_CURVE ( 'NONE', #6593, #14525, #7299, .T. ) ;
#5637=FACE_OUTER_BOUND ( 'NONE', #12030, .T. ) ;
#5641=EDGE_LOOP ( 'NONE', ( #20856, #6335, #176, #12785 ) ) ;
#5645=CARTESIAN_POINT ( 'NONE',  ( 28.97711086133420366, 32.54502000000000095, -10.31874999999999964 ) ) ;
#5658=CIRCLE ( 'NONE', #20471, 1.984374999999998890 ) ;
#5660=DIRECTION ( 'NONE',  ( -0.2868778675745011220, 0.000000000000000000, -0.9579671649362033747 ) ) ;
#5670=AXIS2_PLACEMENT_3D ( 'NONE', #5703, #12572, #14243 ) ;
#5674=VERTEX_POINT ( 'NONE', #9157 ) ;
#5680=VECTOR ( 'NONE', #14902, 1000.000000000000000 ) ;
#5683=ADVANCED_FACE ( 'NONE', ( #11051 ), #19439, .F. ) ;
#5684=CIRCLE ( 'NONE', #6735, 3.175000000000000711 ) ;
#5685=AXIS2_PLACEMENT_3D ( 'NONE', #3608, #280, #3394 ) ;
#5701=ORIENTED_EDGE ( 'NONE', *, *, #5346, .T. ) ;
#5703=CARTESIAN_POINT ( 'NONE',  ( -29.36874999999999858, 1.983739999999999837, 8.731885000000000119 ) ) ;
#5708=EDGE_CURVE ( 'NONE', #13402, #15989, #14529, .T. ) ;
#5719=AXIS2_PLACEMENT_3D ( 'NONE', #17605, #12420, #1007 ) ;
#5739=VERTEX_POINT ( 'NONE', #4853 ) ;
#5751=CARTESIAN_POINT ( 'NONE',  ( 18.65312499999999929, 30.56064500000000095, 5.159374999999999822 ) ) ;
#5752=AXIS2_PLACEMENT_3D ( 'NONE', #9923, #13374, #3309 ) ;
#5759=ORIENTED_EDGE ( 'NONE', *, *, #5859, .F. ) ;
#5761=CARTESIAN_POINT ( 'NONE',  ( 26.59062499999999929, 5.953125000000000000, 8.731249999999999289 ) ) ;
#5767=ADVANCED_FACE ( 'NONE', ( #1418 ), #13165, .T. ) ;
#5768=EDGE_CURVE ( 'NONE', #9142, #2020, #4669, .T. ) ;
#5772=CARTESIAN_POINT ( 'NONE',  ( -2.256261688646920227, 22.62314500000000095, -0.3933872460174320240 ) ) ;
#5778=CYLINDRICAL_SURFACE ( 'NONE', #5719, 9.524999999999998579 ) ;
#5793=EDGE_CURVE ( 'NONE', #1101, #19328, #9709, .T. ) ;
#5801=CYLINDRICAL_SURFACE ( 'NONE', #4742, 0.3962399999999998146 ) ;
#5804=DIRECTION ( 'NONE',  ( 0.000000000000000000, 0.000000000000000000, 1.000000000000000000 ) ) ;
#5805=ORIENTED_EDGE ( 'NONE', *, *, #16191, .T. ) ;
#5815=ORIENTED_EDGE ( 'NONE', *, *, #641, .T. ) ;
#5829=CARTESIAN_POINT ( 'NONE',  ( -1.880134707694870011, 12.30439499999999953, 7.779750394130780400 ) ) ;
#5831=ORIENTED_EDGE ( 'NONE', *, *, #7365, .T. ) ;
#5841=CARTESIAN_POINT ( 'NONE',  ( 26.59062499999999929, 5.953125000000000000, 10.71562499999999929 ) ) ;
#5850=ORIENTED_EDGE ( 'NONE', *, *, #15998, .T. ) ;
#5859=EDGE_CURVE ( 'NONE', #7283, #14216, #10680, .T. ) ;
#5863=EDGE_CURVE ( 'NONE', #13820, #7283, #13276, .T. ) ;
#5873=CARTESIAN_POINT ( 'NONE',  ( 24.60624999999999929, 16.27314499999999953, 8.731249999999999289 ) ) ;
#5876=EDGE_CURVE ( 'NONE', #7268, #9462, #4427, .T. ) ;
#5878=EDGE_CURVE ( 'NONE', #8651, #7667, #11594, .T. ) ;
#5883=CARTESIAN_POINT ( 'NONE',  ( 26.34068084182479907, 1.140633240613131871, 10.52776784000260157 ) ) ;
#5887=ORIENTED_EDGE ( 'NONE', *, *, #14248, .F. ) ;
#5888=CARTESIAN_POINT ( 'NONE',  ( 36.51250000000000284, 0.000000000000000000, -10.31875000000000142 ) ) ;
#5895=CARTESIAN_POINT ( 'NONE',  ( 71.03963378001139972, 1.984375000000000000, -10.54138470677948014 ) ) ;
#5898=EDGE_CURVE ( 'NONE', #21060, #9547, #6397, .T. ) ;
#5902=ORIENTED_EDGE ( 'NONE', *, *, #10301, .F. ) ;
#5919=DIRECTION ( 'NONE',  ( 0.2868778675745004558, 0.000000000000000000, 0.9579671649362035968 ) ) ;
#5921=EDGE_CURVE ( 'NONE', #17008, #1449, #13868, .T. ) ;
#5923=VERTEX_POINT ( 'NONE', #3311 ) ;
#5926=DIRECTION ( 'NONE',  ( -0.2868778675745010664, 0.000000000000000000, -0.9579671649362032637 ) ) ;
#5932=ORIENTED_EDGE ( 'NONE', *, *, #7853, .T. ) ;
#5936=ORIENTED_EDGE ( 'NONE', *, *, #14597, .F. ) ;
#5948=DIRECTION ( 'NONE',  ( 0.000000000000000000, -1.000000000000000000, 0.000000000000000000 ) ) ;
#5951=CARTESIAN_POINT ( 'NONE',  ( 21.43124999999999858, 16.27314499999999953, 8.731249999999999289 ) ) ;
#5952=ORIENTED_EDGE ( 'NONE', *, *, #20286, .T. ) ;
#5953=VERTEX_POINT ( 'NONE', #20083 ) ;
#5958=ORIENTED_EDGE ( 'NONE', *, *, #4769, .F. ) ;
#5972=ADVANCED_FACE ( 'NONE', ( #16791, #20196, #10251, #5066, #21758 ), #17115, .F. ) ;
#5978=PLANE ( 'NONE',  #21243 ) ;
#5983=LINE ( 'NONE', #8302, #7824 ) ;
#5987=CARTESIAN_POINT ( 'NONE',  ( 21.94726064351640105, 0.7124538231385260101, 10.25520621805301857 ) ) ;
#5990=DIRECTION ( 'NONE',  ( 0.000000000000000000, 0.000000000000000000, -1.000000000000000000 ) ) ;
#5991=ORIENTED_EDGE ( 'NONE', *, *, #12328, .T. ) ;
#6001=DIRECTION ( 'NONE',  ( -1.000000000000000000, 0.000000000000000000, 0.000000000000000000 ) ) ;
#6009=FACE_OUTER_BOUND ( 'NONE', #4581, .T. ) ;
#6015=CARTESIAN_POINT ( 'NONE',  ( 30.33489826846160398, 32.54502000000000095, -2.417033907079745525 ) ) ;
#6021=CARTESIAN_POINT ( 'NONE',  ( 5.447351731530780228, 32.54502000000000095, 0.8930339070797439494 ) ) ;
#6023=ORIENTED_EDGE ( 'NONE', *, *, #7365, .F. ) ;
#6029=VECTOR ( 'NONE', #14501, 1000.000000000000000 ) ;
#6036=CARTESIAN_POINT ( 'NONE',  ( 29.36874999999999858, 0.000000000000000000, -10.31874999999999964 ) ) ;
#6049=AXIS2_PLACEMENT_3D ( 'NONE', #109, #5093, #11731 ) ;
#6050=VERTEX_POINT ( 'NONE', #19625 ) ;
#6054=VERTEX_POINT ( 'NONE', #16447 ) ;
#6058=DIRECTION ( 'NONE',  ( -0.9579671649362033747, 0.000000000000000000, 0.2868778675745011220 ) ) ;
#6060=CARTESIAN_POINT ( 'NONE',  ( -20.63749999999999929, 16.27314499999999953, 10.71562499999999929 ) ) ;
#6065=CARTESIAN_POINT ( 'NONE',  ( 46.03750000000000142, 1.984375000000000000, -10.31874999999999964 ) ) ;
#6088=CARTESIAN_POINT ( 'NONE',  ( 29.19635173153840313, 32.54502000000000095, -6.218966092919240296 ) ) ;
#6094=DIRECTION ( 'NONE',  ( 1.000000000000000000, 0.000000000000000000, 0.000000000000000000 ) ) ;
#6097=VERTEX_POINT ( 'NONE', #20154 ) ;
#6099=AXIS2_PLACEMENT_3D ( 'NONE', #15, #6765, #13641 ) ;
#6102=CARTESIAN_POINT ( 'NONE',  ( 27.72321311043520353, 1.355051563794170022, 10.61353820125299841 ) ) ;
#6110=EDGE_CURVE ( 'NONE', #4736, #7142, #18741, .T. ) ;
#6121=AXIS2_PLACEMENT_3D ( 'NONE', #14763, #21469, #19922 ) ;
#6127=ORIENTED_EDGE ( 'NONE', *, *, #15590, .T. ) ;
#6130=VECTOR ( 'NONE', #17318, 1000.000000000000000 ) ;
#6138=CARTESIAN_POINT ( 'NONE',  ( 30.33489826846160398, 32.54502000000000095, -2.417033907079745525 ) ) ;
#6140=EDGE_CURVE ( 'NONE', #18115, #2722, #12408, .T. ) ;
#6143=VECTOR ( 'NONE', #10823, 1000.000000000000000 ) ;
#6155=DIRECTION ( 'NONE',  ( -0.08192867786951699149, 0.000000000000000000, -0.9966381950048638361 ) ) ;
#6160=EDGE_CURVE ( 'NONE', #17319, #8651, #4825, .T. ) ;
#6164=VERTEX_POINT ( 'NONE', #6358 ) ;
#6166=ORIENTED_EDGE ( 'NONE', *, *, #17405, .F. ) ;
#6175=DIRECTION ( 'NONE',  ( 1.000000000000000000, 0.000000000000000000, 0.000000000000000000 ) ) ;
#6180=DIRECTION ( 'NONE',  ( 0.000000000000000000, -1.000000000000000000, 0.000000000000000000 ) ) ;
#6183=EDGE_CURVE ( 'NONE', #3518, #20164, #8343, .T. ) ;
#6189=ORIENTED_EDGE ( 'NONE', *, *, #319, .T. ) ;
#6190=AXIS2_PLACEMENT_3D ( 'NONE', #5257, #4848, #21752 ) ;
#6196=CARTESIAN_POINT ( 'NONE',  ( -17.46249999999999858, 32.54502000000000095, 0.000000000000000000 ) ) ;
#6201=CARTESIAN_POINT ( 'NONE',  ( 26.59062499999999929, 26.59189500000000095, 8.731249999999999289 ) ) ;
#6204=VERTEX_POINT ( 'NONE', #16648 ) ;
#6206=EDGE_CURVE ( 'NONE', #15542, #11564, #21729, .T. ) ;
#6214=EDGE_LOOP ( 'NONE', ( #1917, #16429, #16272, #7308, #2969 ) ) ;
#6218=EDGE_LOOP ( 'NONE', ( #15211, #20520, #2063, #9799, #9801 ) ) ;
#6221=DIRECTION ( 'NONE',  ( -0.2868778675745008999, 0.000000000000000000, -0.9579671649362034858 ) ) ;
#6226=LINE ( 'NONE', #21370, #10438 ) ;
#6236=CIRCLE ( 'NONE', #239, 3.175000000000000711 ) ;
#6238=CARTESIAN_POINT ( 'NONE',  ( 23.41562500000000213, 32.54502000000000095, 5.159374999999999822 ) ) ;
#6241=DIRECTION ( 'NONE',  ( 0.000000000000000000, -1.000000000000000000, 0.000000000000000000 ) ) ;
#6248=EDGE_CURVE ( 'NONE', #2429, #12596, #2159, .T. ) ;
#6256=ADVANCED_FACE ( 'NONE', ( #16639 ), #16754, .T. ) ;
#6274=DIRECTION ( 'NONE',  ( 0.000000000000000000, 0.000000000000000000, -1.000000000000000000 ) ) ;
#6276=VECTOR ( 'NONE', #12521, 1000.000000000000000 ) ;
#6280=CARTESIAN_POINT ( 'NONE',  ( 26.59062499999999929, 2.380615000000000148, 8.731249999999999289 ) ) ;
#6290=DIRECTION ( 'NONE',  ( 0.000000000000000000, 1.000000000000000000, 0.000000000000000000 ) ) ;
#6294=EDGE_CURVE ( 'NONE', #9547, #8281, #15206, .T. ) ;
#6299=DIRECTION ( 'NONE',  ( 0.000000000000000000, 0.000000000000000000, 1.000000000000000000 ) ) ;
#6310=VERTEX_POINT ( 'NONE', #20255 ) ;
#6316=CARTESIAN_POINT ( 'NONE',  ( 26.66313208013160008, 1.184654662339226006, 10.54777226219331965 ) ) ;
#6322=ADVANCED_FACE ( 'NONE', ( #4908 ), #9872, .F. ) ;
#6324=CARTESIAN_POINT ( 'NONE',  ( 0.05261182704408059324, 23.41816500000000190, 7.316601101023040066 ) ) ;
#6328=CARTESIAN_POINT ( 'NONE',  ( -1.345424459097947834, 20.24316500000000119, 2.648158502653860324 ) ) ;
#6335=ORIENTED_EDGE ( 'NONE', *, *, #3459, .T. ) ;
#6339=ORIENTED_EDGE ( 'NONE', *, *, #4097, .F. ) ;
#6350=ORIENTED_EDGE ( 'NONE', *, *, #14654, .F. ) ;
#6356=ORIENTED_EDGE ( 'NONE', *, *, #7613, .T. ) ;
#6358=CARTESIAN_POINT ( 'NONE',  ( 2.063750000000000195, 24.21318500000000284, 10.71562499999999929 ) ) ;
#6375=EDGE_CURVE ( 'NONE', #8773, #3294, #6895, .T. ) ;
#6388=PLANE ( 'NONE',  #1900 ) ;
#6389=AXIS2_PLACEMENT_3D ( 'NONE', #8230, #13435, #150 ) ;
#6390=CARTESIAN_POINT ( 'NONE',  ( 66.03921914090641110, 0.000000000000000000, -10.93409647675949969 ) ) ;
#6397=LINE ( 'NONE', #11487, #377 ) ;
#6399=ORIENTED_EDGE ( 'NONE', *, *, #17925, .T. ) ;
#6403=ORIENTED_EDGE ( 'NONE', *, *, #764, .F. ) ;
#6407=LINE ( 'NONE', #1539, #5309 ) ;
#6409=AXIS2_PLACEMENT_3D ( 'NONE', #9413, #15854, #4117 ) ;
#6412=AXIS2_PLACEMENT_3D ( 'NONE', #6743, #1441, #11616 ) ;
#6423=DIRECTION ( 'NONE',  ( 1.000000000000000000, 0.000000000000000000, 0.000000000000000000 ) ) ;
#6431=EDGE_CURVE ( 'NONE', #9031, #14393, #3915, .T. ) ;
#6440=DIRECTION ( 'NONE',  ( 0.000000000000000000, 1.000000000000000000, 0.000000000000000000 ) ) ;
#6441=VECTOR ( 'NONE', #15137, 1000.000000000000000 ) ;
#6445=CARTESIAN_POINT ( 'NONE',  ( 2.063750000000000195, 24.21318500000000284, 8.731249999999999289 ) ) ;
#6454=DIRECTION ( 'NONE',  ( 0.000000000000000000, 1.000000000000000000, 0.000000000000000000 ) ) ;
#6460=VERTEX_POINT ( 'NONE', #17515 ) ;
#6463=DIRECTION ( 'NONE',  ( 0.000000000000000000, 0.000000000000000000, -1.000000000000000000 ) ) ;
#6464=CARTESIAN_POINT ( 'NONE',  ( -23.01875000000000071, 30.56064500000000095, -3.968750000000000000 ) ) ;
#6470=CARTESIAN_POINT ( 'NONE',  ( -29.36874999999999858, 1.984375000000000000, 8.731249999999999289 ) ) ;
#6487=DIRECTION ( 'NONE',  ( 0.1831666983862991482, 0.000000000000000000, -0.9830818687180954418 ) ) ;
#6501=CYLINDRICAL_SURFACE ( 'NONE', #14982, 0.3962400000000008138 ) ;
#6503=VECTOR ( 'NONE', #13046, 1000.000000000000000 ) ;
#6515=CARTESIAN_POINT ( 'NONE',  ( -20.63749999999999929, 16.27314499999999953, 8.731249999999999289 ) ) ;
#6518=ORIENTED_EDGE ( 'NONE', *, *, #20540, .F. ) ;
#6522=CARTESIAN_POINT ( 'NONE',  ( 6.016625000000000334, 32.54502000000000095, 2.794000000000000039 ) ) ;
#6525=ORIENTED_EDGE ( 'NONE', *, *, #9623, .T. ) ;
#6526=DIRECTION ( 'NONE',  ( 0.000000000000000000, 1.000000000000000000, 0.000000000000000000 ) ) ;
#6539=CARTESIAN_POINT ( 'NONE',  ( 67.40134256979101224, 30.56064500000000095, -13.70358117861468017 ) ) ;
#6542=ADVANCED_FACE ( 'NONE', ( #12765 ), #9316, .F. ) ;
#6550=( NAMED_UNIT ( * ) PLANE_ANGLE_UNIT ( ) SI_UNIT ( $, .RADIAN. ) );
#6553=EDGE_CURVE ( 'NONE', #12688, #19126, #3227, .T. ) ;
#6556=CARTESIAN_POINT ( 'NONE',  ( 66.03921914090641110, 0.000000000000000000, -10.93409647675949969 ) ) ;
#6557=EDGE_CURVE ( 'NONE', #8141, #11451, #16089, .T. ) ;
#6561=DIRECTION ( 'NONE',  ( 0.000000000000000000, -1.000000000000000000, 0.000000000000000000 ) ) ;
#6566=CYLINDRICAL_SURFACE ( 'NONE', #11180, 9.524999999999998579 ) ;
#6573=( LENGTH_UNIT ( ) NAMED_UNIT ( * ) SI_UNIT ( .MILLI., .METRE. ) );
#6574=DIRECTION ( 'NONE',  ( 0.9579671649362034858, 0.000000000000000000, -0.2868778675745011220 ) ) ;
#6576=ORIENTED_EDGE ( 'NONE', *, *, #15998, .F. ) ;
#6582=ADVANCED_FACE ( 'NONE', ( #21359 ), #12650, .T. ) ;
#6583=CARTESIAN_POINT ( 'NONE',  ( 66.87634738983680904, 30.56064500000000095, 3.497859541731999755 ) ) ;
#6593=VERTEX_POINT ( 'NONE', #9532 ) ;
#6603=EDGE_CURVE ( 'NONE', #7901, #3268, #12985, .T. ) ;
#6608=EDGE_LOOP ( 'NONE', ( #10510, #10284, #4936, #17903 ) ) ;
#6609=CARTESIAN_POINT ( 'NONE',  ( 66.87634738983680904, 0.000000000000000000, 3.497859541731999755 ) ) ;
#6618=FACE_OUTER_BOUND ( 'NONE', #501, .T. ) ;
#6622=EDGE_CURVE ( 'NONE', #18576, #7181, #6709, .T. ) ;
#6627=VERTEX_POINT ( 'NONE', #18055 ) ;
#6635=MANIFOLD_SOLID_BREP ( 'Stock-MAS-676-1', #9939 ) ;
#6641=DIRECTION ( 'NONE',  ( -1.000000000000000000, 0.000000000000000000, 0.000000000000000000 ) ) ;
#6642=DIRECTION ( 'NONE',  ( -1.000000000000000000, 0.000000000000000000, 0.000000000000000000 ) ) ;
#6645=PLANE ( 'NONE',  #18862 ) ;
#6650=EDGE_CURVE ( 'NONE', #12037, #4819, #16825, .T. ) ;
#6658=CARTESIAN_POINT ( 'NONE',  ( 36.51250000000000284, 1.984375000000000000, -10.31875000000000142 ) ) ;
#6664=AXIS2_PLACEMENT_3D ( 'NONE', #17846, #14101, #2581 ) ;
#6670=FACE_OUTER_BOUND ( 'NONE', #12910, .T. ) ;
#6685=AXIS2_PLACEMENT_3D ( 'NONE', #12991, #2916, #21582 ) ;
#6691=ORIENTED_EDGE ( 'NONE', *, *, #7853, .F. ) ;
#6704=AXIS2_PLACEMENT_3D ( 'NONE', #17160, #3356, #18692 ) ;
#6709=CIRCLE ( 'NONE', #4956, 0.7950200000000007261 ) ;
#6719=VERTEX_POINT ( 'NONE', #14977 ) ;
#6729=EDGE_CURVE ( 'NONE', #2932, #11624, #6874, .T. ) ;
#6730=CARTESIAN_POINT ( 'NONE',  ( -12.30312499704650087, 1.984216250000054860, 10.71562498306123956 ) ) ;
#6735=AXIS2_PLACEMENT_3D ( 'NONE', #20577, #17506, #10648 ) ;
#6737=LINE ( 'NONE', #5283, #20596 ) ;
#6743=CARTESIAN_POINT ( 'NONE',  ( 65.67421548912699336, 0.000000000000000000, -10.93409647675949969 ) ) ;
#6747=LINE ( 'NONE', #21567, #13739 ) ;
#6762=ADVANCED_FACE ( 'NONE', ( #18687 ), #13205, .F. ) ;
#6765=DIRECTION ( 'NONE',  ( 0.000000000000000000, 1.000000000000000000, 0.000000000000000000 ) ) ;
#6768=LINE ( 'NONE', #11864, #10803 ) ;
#6773=VECTOR ( 'NONE', #656, 1000.000000000000000 ) ;
#6780=DIRECTION ( 'NONE',  ( 0.000000000000000000, 0.000000000000000000, -1.000000000000000000 ) ) ;
#6781=EDGE_CURVE ( 'NONE', #4180, #15382, #17037, .T. ) ;
#6787=DIRECTION ( 'NONE',  ( -0.2868778675745011220, 0.000000000000000000, -0.9579671649362033747 ) ) ;
#6806=ORIENTED_EDGE ( 'NONE', *, *, #9240, .T. ) ;
#6807=ORIENTED_EDGE ( 'NONE', *, *, #17760, .F. ) ;
#6808=FACE_OUTER_BOUND ( 'NONE', #3527, .T. ) ;
#6814=VERTEX_POINT ( 'NONE', #10625 ) ;
#6823=LINE ( 'NONE', #10362, #20531 ) ;
#6828=EDGE_CURVE ( 'NONE', #11451, #13089, #4256, .T. ) ;
#6829=CARTESIAN_POINT ( 'NONE',  ( 26.59062499999999929, 5.953125000000000000, 8.731249999999999289 ) ) ;
#6833=PLANE ( 'NONE',  #7151 ) ;
#6838=AXIS2_PLACEMENT_3D ( 'NONE', #14659, #2920, #13210 ) ;
#6846=CARTESIAN_POINT ( 'NONE',  ( 49.09065990372640442, 0.000000000000000000, -26.70549589918839928 ) ) ;
#6847=ORIENTED_EDGE ( 'NONE', *, *, #2240, .F. ) ;
#6851=CARTESIAN_POINT ( 'NONE',  ( 29.37324403177899868, 1.984375000000000000, -10.70578951775076071 ) ) ;
#6857=ORIENTED_EDGE ( 'NONE', *, *, #843, .T. ) ;
#6864=EDGE_LOOP ( 'NONE', ( #4856, #11736, #16245, #6691, #16579, #1399 ) ) ;
#6874=LINE ( 'NONE', #13311, #17674 ) ;
#6876=LINE ( 'NONE', #13525, #161 ) ;
#6879=CIRCLE ( 'NONE', #19239, 22.02656249999999005 ) ;
#6895=LINE ( 'NONE', #20358, #739 ) ;
#6904=EDGE_CURVE ( 'NONE', #7279, #19333, #3777, .T. ) ;
#6913=ORIENTED_EDGE ( 'NONE', *, *, #19245, .F. ) ;
#6915=FACE_OUTER_BOUND ( 'NONE', #15673, .T. ) ;
#6923=DIRECTION ( 'NONE',  ( 0.000000000000000000, 1.000000000000000000, 0.000000000000000000 ) ) ;
#6932=CARTESIAN_POINT ( 'NONE',  ( 1.268730000000000135, 9.129395000000000593, 10.65596716962832069 ) ) ;
#6957=CIRCLE ( 'NONE', #3430, 0.3962399999999998146 ) ;
#6958=ORIENTED_EDGE ( 'NONE', *, *, #14628, .F. ) ;
#6963=EDGE_LOOP ( 'NONE', ( #11701, #12234, #13162, #19409, #3322, #19301 ) ) ;
#6973=EDGE_CURVE ( 'NONE', #11160, #19865, #15927, .T. ) ;
#6998=DIRECTION ( 'NONE',  ( 1.000000000000000000, 0.000000000000000000, 0.000000000000000000 ) ) ;
#7013=VERTEX_POINT ( 'NONE', #9168 ) ;
#7018=CIRCLE ( 'NONE', #13042, 0.3962399999999988154 ) ;
#7025=EDGE_CURVE ( 'NONE', #13038, #21568, #21109, .T. ) ;
#7028=ORIENTED_EDGE ( 'NONE', *, *, #7631, .F. ) ;
#7031=DIRECTION ( 'NONE',  ( -0.2868778675745008999, 0.000000000000000000, -0.9579671649362034858 ) ) ;
#7036=DIRECTION ( 'NONE',  ( 1.000000000000000000, 0.000000000000000000, 0.000000000000000000 ) ) ;
#7037=EDGE_LOOP ( 'NONE', ( #14220, #695, #11513, #4850 ) ) ;
#7045=DIRECTION ( 'NONE',  ( 0.000000000000000000, 0.000000000000000000, -1.000000000000000000 ) ) ;
#7052=ORIENTED_EDGE ( 'NONE', *, *, #705, .F. ) ;
#7061=DIRECTION ( 'NONE',  ( -0.08192867786951699149, 0.000000000000000000, -0.9966381950048638361 ) ) ;
#7064=DIRECTION ( 'NONE',  ( 0.000000000000000000, 1.000000000000000000, 0.000000000000000000 ) ) ;
#7066=DIRECTION ( 'NONE',  ( 1.000000000000000000, 0.000000000000000000, 0.000000000000000000 ) ) ;
#7087=DIRECTION ( 'NONE',  ( 1.000000000000000000, 0.000000000000000000, 0.000000000000000000 ) ) ;
#7092=EDGE_CURVE ( 'NONE', #20045, #8589, #16060, .T. ) ;
#7103=DIRECTION ( 'NONE',  ( -1.000000000000000000, 0.000000000000000000, 0.000000000000000000 ) ) ;
#7115=DIRECTION ( 'NONE',  ( 0.000000000000000000, 1.000000000000000000, 0.000000000000000000 ) ) ;
#7117=EDGE_LOOP ( 'NONE', ( #7390, #9991, #3172, #8539 ) ) ;
#7121=DIRECTION ( 'NONE',  ( 1.000000000000000000, 0.000000000000000000, 0.000000000000000000 ) ) ;
#7134=DIRECTION ( 'NONE',  ( 0.000000000000000000, -1.000000000000000000, 0.000000000000000000 ) ) ;
#7142=VERTEX_POINT ( 'NONE', #16378 ) ;
#7151=AXIS2_PLACEMENT_3D ( 'NONE', #3408, #11816, #13375 ) ;
#7167=LINE ( 'NONE', #14258, #3646 ) ;
#7181=VERTEX_POINT ( 'NONE', #16590 ) ;
#7183=AXIS2_PLACEMENT_3D ( 'NONE', #16736, #4891, #243 ) ;
#7184=ORIENTED_EDGE ( 'NONE', *, *, #5921, .T. ) ;
#7193=EDGE_CURVE ( 'NONE', #13038, #395, #7961, .T. ) ;
#7194=FACE_BOUND ( 'NONE', #11474, .T. ) ;
#7195=EDGE_CURVE ( 'NONE', #12892, #13849, #729, .T. ) ;
#7200=DIRECTION ( 'NONE',  ( 0.000000000000000000, 0.000000000000000000, 1.000000000000000000 ) ) ;
#7204=AXIS2_PLACEMENT_3D ( 'NONE', #3235, #1458, #16616 ) ;
#7205=CARTESIAN_POINT ( 'NONE',  ( 29.76562500000000000, 32.54502000000000095, -4.317999999999999616 ) ) ;
#7217=EDGE_CURVE ( 'NONE', #19328, #6310, #16698, .T. ) ;
#7224=EDGE_CURVE ( 'NONE', #12892, #19746, #21662, .T. ) ;
#7225=EDGE_CURVE ( 'NONE', #10798, #12065, #1639, .T. ) ;
#7234=ORIENTED_EDGE ( 'NONE', *, *, #7432, .F. ) ;
#7238=VECTOR ( 'NONE', #1486, 1000.000000000000227 ) ;
#7242=EDGE_CURVE ( 'NONE', #7810, #21532, #21437, .T. ) ;
#7263=ORIENTED_EDGE ( 'NONE', *, *, #18069, .F. ) ;
#7265=EDGE_CURVE ( 'NONE', #9462, #777, #6407, .T. ) ;
#7266=ADVANCED_FACE ( 'NONE', ( #11603 ), #2996, .F. ) ;
#7268=VERTEX_POINT ( 'NONE', #6730 ) ;
#7277=DIRECTION ( 'NONE',  ( 0.000000000000000000, 1.000000000000000000, 0.000000000000000000 ) ) ;
#7279=VERTEX_POINT ( 'NONE', #13176 ) ;
#7280=ORIENTED_EDGE ( 'NONE', *, *, #11801, .F. ) ;
#7283=VERTEX_POINT ( 'NONE', #18558 ) ;
#7289=ADVANCED_FACE ( 'NONE', ( #3419 ), #18339, .F. ) ;
#7290=ORIENTED_EDGE ( 'NONE', *, *, #17344, .F. ) ;
#7291=CARTESIAN_POINT ( 'NONE',  ( 15.58268548097005102, 0.3514302678472279728, 9.860356909081639643 ) ) ;
#7292=CARTESIAN_POINT ( 'NONE',  ( 66.03921914090641110, 30.56064500000000095, -10.93409647675949969 ) ) ;
#7293=CARTESIAN_POINT ( 'NONE',  ( 36.51250000000000284, 0.000000000000000000, -10.31875000000000142 ) ) ;
#7299=LINE ( 'NONE', #19229, #18772 ) ;
#7308=ORIENTED_EDGE ( 'NONE', *, *, #15817, .T. ) ;
#7323=CYLINDRICAL_SURFACE ( 'NONE', #16706, 0.3962399999999975386 ) ;
#7326=FACE_OUTER_BOUND ( 'NONE', #5501, .T. ) ;
#7338=ADVANCED_FACE ( 'NONE', ( #6618 ), #11392, .F. ) ;
#7340=EDGE_CURVE ( 'NONE', #12596, #14993, #9721, .T. ) ;
#7341=DIRECTION ( 'NONE',  ( 0.9579671649362034858, 0.000000000000000000, -0.2868778675745011220 ) ) ;
#7342=EDGE_LOOP ( 'NONE', ( #17459, #11821, #20408, #18887 ) ) ;
#7346=CIRCLE ( 'NONE', #13719, 6.349999999999999645 ) ;
#7352=EDGE_CURVE ( 'NONE', #9795, #3518, #2850, .T. ) ;
#7354=VERTEX_POINT ( 'NONE', #4960 ) ;
#7362=CARTESIAN_POINT ( 'NONE',  ( 1.874333784495441968, 8.854522058277447982, 8.730299172444558664 ) ) ;
#7365=EDGE_CURVE ( 'NONE', #4077, #17862, #11715, .T. ) ;
#7366=DIRECTION ( 'NONE',  ( -0.1831666983862943188, 0.000000000000000000, 0.9830818687180962190 ) ) ;
#7372=AXIS2_PLACEMENT_3D ( 'NONE', #19440, #17691, #4314 ) ;
#7374=DIRECTION ( 'NONE',  ( 0.000000000000000000, 1.000000000000000000, 0.000000000000000000 ) ) ;
#7376=EDGE_CURVE ( 'NONE', #8589, #10232, #4276, .T. ) ;
#7378=DIRECTION ( 'NONE',  ( 0.3850029901312932989, 0.000000000000000000, -0.9229153252546862252 ) ) ;
#7379=CARTESIAN_POINT ( 'NONE',  ( 70.64340948846358970, 1.984375000000000000, -10.93409647675949969 ) ) ;
#7389=VERTEX_POINT ( 'NONE', #9117 ) ;
#7390=ORIENTED_EDGE ( 'NONE', *, *, #7769, .F. ) ;
#7395=AXIS2_PLACEMENT_3D ( 'NONE', #19914, #19801, #4677 ) ;
#7399=ORIENTED_EDGE ( 'NONE', *, *, #16959, .T. ) ;
#7402=DIRECTION ( 'NONE',  ( 0.000000000000000000, 1.000000000000000000, 0.000000000000000000 ) ) ;
#7404=EDGE_CURVE ( 'NONE', #1876, #1202, #2389, .T. ) ;
#7408=DIRECTION ( 'NONE',  ( -0.9579671649362032637, 0.000000000000000000, 0.2868778675745010664 ) ) ;
#7417=CIRCLE ( 'NONE', #10234, 1.984374999999999112 ) ;
#7429=DIRECTION ( 'NONE',  ( -0.08192867786951699149, 0.000000000000000000, -0.9966381950048638361 ) ) ;
#7432=EDGE_CURVE ( 'NONE', #218, #19957, #14171, .T. ) ;
#7445=AXIS2_PLACEMENT_3D ( 'NONE', #2810, #6454, #16315 ) ;
#7450=DIRECTION ( 'NONE',  ( 0.000000000000000000, 1.000000000000000000, 0.000000000000000000 ) ) ;
#7454=CARTESIAN_POINT ( 'NONE',  ( 46.03750000000000142, 30.56064500000000095, -10.31874999999999964 ) ) ;
#7473=VECTOR ( 'NONE', #1239, 1000.000000000000114 ) ;
#7475=AXIS2_PLACEMENT_3D ( 'NONE', #13305, #18254, #11622 ) ;
#7485=DIRECTION ( 'NONE',  ( 0.2868778675745004558, 0.000000000000000000, 0.9579671649362035968 ) ) ;
#7490=EDGE_CURVE ( 'NONE', #4077, #5219, #13817, .T. ) ;
#7497=PLANE ( 'NONE',  #733 ) ;
#7503=VECTOR ( 'NONE', #20972, 1000.000000000000000 ) ;
#7507=EDGE_CURVE ( 'NONE', #1876, #3944, #2519, .T. ) ;
#7511=CARTESIAN_POINT ( 'NONE',  ( 65.64431122251959039, 30.56064500000000095, -11.29787305743958115 ) ) ;
#7513=CARTESIAN_POINT ( 'NONE',  ( 1.337733264118907694, 23.41816499999999834, 8.634866101730979793 ) ) ;
#7514=DIRECTION ( 'NONE',  ( 0.000000000000000000, 1.000000000000000000, 0.000000000000000000 ) ) ;
#7530=CARTESIAN_POINT ( 'NONE',  ( 46.03750000000000142, 0.000000000000000000, -10.31874999999999964 ) ) ;
#7533=CARTESIAN_POINT ( 'NONE',  ( 65.90927232300019512, 30.56064500000000095, -13.30734117861468135 ) ) ;
#7539=EDGE_CURVE ( 'NONE', #6164, #17225, #8156, .T. ) ;
#7545=LINE ( 'NONE', #21123, #16369 ) ;
#7550=ORIENTED_EDGE ( 'NONE', *, *, #6110, .F. ) ;
#7562=ADVANCED_FACE ( 'NONE', ( #15269 ), #15381, .T. ) ;
#7573=VERTEX_POINT ( 'NONE', #19943 ) ;
#7583=EDGE_LOOP ( 'NONE', ( #2688, #17869 ) ) ;
#7585=AXIS2_PLACEMENT_3D ( 'NONE', #20538, #3533, #8613 ) ;
#7592=ORIENTED_EDGE ( 'NONE', *, *, #7224, .T. ) ;
#7595=CIRCLE ( 'NONE', #18886, 1.984374999999999112 ) ;
#7596=DIRECTION ( 'NONE',  ( 0.000000000000000000, -1.000000000000000000, 0.000000000000000000 ) ) ;
#7602=DIRECTION ( 'NONE',  ( 0.000000000000000000, -1.000000000000000000, 0.000000000000000000 ) ) ;
#7607=ADVANCED_FACE ( 'NONE', ( #13120 ), #19718, .F. ) ;
#7608=ORIENTED_EDGE ( 'NONE', *, *, #5863, .T. ) ;
#7609=ORIENTED_EDGE ( 'NONE', *, *, #8322, .T. ) ;
#7613=EDGE_CURVE ( 'NONE', #1856, #15382, #11339, .T. ) ;
#7631=EDGE_CURVE ( 'NONE', #15924, #20164, #16537, .T. ) ;
#7636=CARTESIAN_POINT ( 'NONE',  ( -2.028188046367890074, 9.129395000000000593, 0.3682158094503220069 ) ) ;
#7639=ADVANCED_FACE ( 'NONE', ( #11005, #9449 ), #14562, .F. ) ;
#7641=CARTESIAN_POINT ( 'NONE',  ( -3.929154139288399961, 9.129395000000000593, 0.9374890779182719625 ) ) ;
#7649=DIRECTION ( 'NONE',  ( 0.000000000000000000, -1.000000000000000000, 0.000000000000000000 ) ) ;
#7662=FACE_OUTER_BOUND ( 'NONE', #14267, .T. ) ;
#7667=VERTEX_POINT ( 'NONE', #14782 ) ;
#7675=CARTESIAN_POINT ( 'NONE',  ( 1.268730000000000135, 24.21318500000000284, 69.04070710741299877 ) ) ;
#7681=ORIENTED_EDGE ( 'NONE', *, *, #5768, .F. ) ;
#7685=DIRECTION ( 'NONE',  ( -0.7776383362760926898, 0.000000000000000000, 0.6287118719681938916 ) ) ;
#7692=CARTESIAN_POINT ( 'NONE',  ( -4.157227781567939928, 9.924415000000001541, 0.1758860224507720060 ) ) ;
#7703=CARTESIAN_POINT ( 'NONE',  ( -29.36874999999999858, 1.983739999999999837, 10.71562499999999929 ) ) ;
#7705=VERTEX_POINT ( 'NONE', #2716 ) ;
#7706=EDGE_CURVE ( 'NONE', #9189, #3005, #2823, .T. ) ;
#7707=AXIS2_PLACEMENT_3D ( 'NONE', #3723, #3612, #5369 ) ;
#7711=ORIENTED_EDGE ( 'NONE', *, *, #11479, .T. ) ;
#7714=VERTEX_POINT ( 'NONE', #21281 ) ;
#7716=ORIENTED_EDGE ( 'NONE', *, *, #10174, .T. ) ;
#7729=VECTOR ( 'NONE', #301, 1000.000000000000000 ) ;
#7730=ORIENTED_EDGE ( 'NONE', *, *, #10267, .T. ) ;
#7731=ORIENTED_EDGE ( 'NONE', *, *, #4721, .T. ) ;
#7734=EDGE_CURVE ( 'NONE', #2217, #1202, #19799, .T. ) ;
#7735=LINE ( 'NONE', #9606, #2363 ) ;
#7739=EDGE_LOOP ( 'NONE', ( #16969, #15017, #17119, #12216, #9476, #6518, #4147, #17345, #765, #15243, #1162, #11983, #16920, #3994, #20719, #20363, #15810, #1067, #9963, #197, #7952, #15890, #3036, #12433, #5519, #18852, #17783 ) ) ;
#7740=CARTESIAN_POINT ( 'NONE',  ( -2.607150795738780058, 0.000000000000000000, 8.731885000000000119 ) ) ;
#7744=AXIS2_PLACEMENT_3D ( 'NONE', #16986, #1839, #8580 ) ;
#7753=DIRECTION ( 'NONE',  ( 0.000000000000000000, -1.000000000000000000, 0.000000000000000000 ) ) ;
#7755=CARTESIAN_POINT ( 'NONE',  ( 1.883521391995739203, 23.69003045368055282, 10.71562500000000107 ) ) ;
#7756=FACE_BOUND ( 'NONE', #4257, .T. ) ;
#7759=PLANE ( 'NONE',  #8873 ) ;
#7760=EDGE_CURVE ( 'NONE', #7279, #13567, #3284, .T. ) ;
#7763=CARTESIAN_POINT ( 'NONE',  ( 25.61392306623480053, 1.050555293943630009, 10.48268080777146061 ) ) ;
#7769=EDGE_CURVE ( 'NONE', #20984, #2328, #15958, .T. ) ;
#7784=ORIENTED_EDGE ( 'NONE', *, *, #7490, .F. ) ;
#7794=CARTESIAN_POINT ( 'NONE',  ( 18.25624999999999787, 16.27314499999999953, 8.731249999999999289 ) ) ;
#7797=LINE ( 'NONE', #21495, #7238 ) ;
#7798=AXIS2_PLACEMENT_3D ( 'NONE', #11344, #15114, #2952 ) ;
#7799=AXIS2_PLACEMENT_3D ( 'NONE', #18450, #13285, #13064 ) ;
#7800=ORIENTED_EDGE ( 'NONE', *, *, #21503, .T. ) ;
#7806=DIRECTION ( 'NONE',  ( 0.000000000000000000, -1.000000000000000000, 0.000000000000000000 ) ) ;
#7810=VERTEX_POINT ( 'NONE', #11236 ) ;
#7811=ORIENTED_EDGE ( 'NONE', *, *, #19425, .F. ) ;
#7812=DIRECTION ( 'NONE',  ( -0.6287118719681975554, 0.000000000000000000, -0.7776383362760898033 ) ) ;
#7823=VECTOR ( 'NONE', #1120, 1000.000000000000000 ) ;
#7824=VECTOR ( 'NONE', #4781, 1000.000000000000000 ) ;
#7827=DIRECTION ( 'NONE',  ( -0.08192867786951699149, 0.000000000000000000, -0.9966381950048638361 ) ) ;
#7844=ORIENTED_EDGE ( 'NONE', *, *, #6729, .F. ) ;
#7852=VECTOR ( 'NONE', #17743, 1000.000000000000000 ) ;
#7853=EDGE_CURVE ( 'NONE', #7714, #8805, #21402, .T. ) ;
#7870=CARTESIAN_POINT ( 'NONE',  ( 27.93851334206399883, 1.396555486991390094, 10.62689512540016068 ) ) ;
#7877=DIRECTION ( 'NONE',  ( 0.9980811434661737147, 0.000000000000000000, 0.06191955310929838502 ) ) ;
#7879=CARTESIAN_POINT ( 'NONE',  ( 21.03437500000000071, 32.54502000000000095, 5.159374999999999822 ) ) ;
#7880=EDGE_CURVE ( 'NONE', #7705, #3294, #21572, .T. ) ;
#7883=EDGE_CURVE ( 'NONE', #1876, #7573, #20499, .T. ) ;
#7891=CIRCLE ( 'NONE', #15687, 1.984374999999999112 ) ;
#7892=CYLINDRICAL_SURFACE ( 'NONE', #12751, 6.349999999999997868 ) ;
#7901=VERTEX_POINT ( 'NONE', #11674 ) ;
#7913=EDGE_CURVE ( 'NONE', #17335, #9687, #9894, .T. ) ;
#7920=ORIENTED_EDGE ( 'NONE', *, *, #21653, .F. ) ;
#7928=CARTESIAN_POINT ( 'NONE',  ( 1.268730000000000135, 9.129395000000000593, 8.609509071587499562 ) ) ;
#7932=VERTEX_POINT ( 'NONE', #18522 ) ;
#7933=EDGE_CURVE ( 'NONE', #7932, #19746, #8494, .T. ) ;
#7941=CARTESIAN_POINT ( 'NONE',  ( -12.30312499999999964, 2.380615000000000148, 8.731249999999999289 ) ) ;
#7942=LINE ( 'NONE', #12831, #1195 ) ;
#7943=DIRECTION ( 'NONE',  ( -0.9966381950048638361, 0.000000000000000000, 0.08192867786951606168 ) ) ;
#7946=CARTESIAN_POINT ( 'NONE',  ( 1.954387715434429795, 9.129395000000000593, 6.745605000000000295 ) ) ;
#7947=CARTESIAN_POINT ( 'NONE',  ( 65.64431122251959039, 1.984375000000000000, -11.29787305743958115 ) ) ;
#7952=ORIENTED_EDGE ( 'NONE', *, *, #468, .F. ) ;
#7961=LINE ( 'NONE', #1427, #3555 ) ;
#7964=AXIS2_PLACEMENT_3D ( 'NONE', #18590, #7103, #1898 ) ;
#7965=DIRECTION ( 'NONE',  ( 0.000000000000000000, 1.000000000000000000, 0.000000000000000000 ) ) ;
#7969=CARTESIAN_POINT ( 'NONE',  ( 54.51779242482700027, 30.56064500000000095, -30.64740209392260084 ) ) ;
#7975=ORIENTED_EDGE ( 'NONE', *, *, #4022, .F. ) ;
#7980=CARTESIAN_POINT ( 'NONE',  ( 29.36887348155339694, 1.984374998761125219, 10.71562877576799977 ) ) ;
#7989=FACE_OUTER_BOUND ( 'NONE', #8790, .T. ) ;
#8002=EDGE_CURVE ( 'NONE', #21819, #3005, #5684, .T. ) ;
#8008=CARTESIAN_POINT ( 'NONE',  ( 46.03750000000000142, 1.984375000000000000, -10.31874999999999964 ) ) ;
#8011=DIRECTION ( 'NONE',  ( 0.8334497143791951279, 0.000000000000000000, 0.5525953072558960066 ) ) ;
#8021=VECTOR ( 'NONE', #4859, 1000.000000000000000 ) ;
#8026=VERTEX_POINT ( 'NONE', #10863 ) ;
#8035=VECTOR ( 'NONE', #12481, 1000.000000000000227 ) ;
#8038=ORIENTED_EDGE ( 'NONE', *, *, #21688, .F. ) ;
#8047=EDGE_CURVE ( 'NONE', #9687, #3268, #5983, .T. ) ;
#8055=ORIENTED_EDGE ( 'NONE', *, *, #16264, .T. ) ;
#8064=VECTOR ( 'NONE', #2390, 1000.000000000000114 ) ;
#8071=CARTESIAN_POINT ( 'NONE',  ( 28.97711086133420366, 32.54502000000000095, -10.31874999999999964 ) ) ;
#8079=CIRCLE ( 'NONE', #20414, 0.3962400000000010358 ) ;
#8084=LINE ( 'NONE', #16506, #14136 ) ;
#8087=CARTESIAN_POINT ( 'NONE',  ( 29.36874999999999858, 22.62187499999999929, 8.731249999999999289 ) ) ;
#8094=PLANE ( 'NONE',  #71 ) ;
#8096=DIRECTION ( 'NONE',  ( 0.6287118719681975554, 0.000000000000000000, 0.7776383362760898033 ) ) ;
#8111=CARTESIAN_POINT ( 'NONE',  ( 6.016625000000000334, 32.54502000000000095, 2.794000000000000039 ) ) ;
#8122=ADVANCED_FACE ( 'NONE', ( #11511 ), #11739, .F. ) ;
#8127=ORIENTED_EDGE ( 'NONE', *, *, #7933, .T. ) ;
#8139=EDGE_LOOP ( 'NONE', ( #11384, #10222, #3195, #15267, #17685, #4245, #12118, #14048, #16046, #8891, #20953, #16817 ) ) ;
#8141=VERTEX_POINT ( 'NONE', #117 ) ;
#8143=EDGE_CURVE ( 'NONE', #12037, #13767, #13625, .T. ) ;
#8144=DIRECTION ( 'NONE',  ( 1.000000000000000000, 0.000000000000000000, 0.000000000000000000 ) ) ;
#8145=EDGE_LOOP ( 'NONE', ( #17933, #3523, #20299, #4644 ) ) ;
#8151=LINE ( 'NONE', #11043, #3601 ) ;
#8154=DIRECTION ( 'NONE',  ( 0.000000000000000000, 1.000000000000000000, 0.000000000000000000 ) ) ;
#8156=CIRCLE ( 'NONE', #1107, 0.7950200000000000600 ) ;
#8159=DIRECTION ( 'NONE',  ( 1.000000000000000000, 0.000000000000000000, 0.000000000000000000 ) ) ;
#8162=DIRECTION ( 'NONE',  ( 0.000000000000000000, -1.000000000000000000, 0.000000000000000000 ) ) ;
#8166=CYLINDRICAL_SURFACE ( 'NONE', #12627, 1.984375000000000888 ) ;
#8169=ORIENTED_EDGE ( 'NONE', *, *, #17650, .T. ) ;
#8170=DIRECTION ( 'NONE',  ( 0.000000000000000000, 1.000000000000000000, 0.000000000000000000 ) ) ;
#8188=DIRECTION ( 'NONE',  ( 0.000000000000000000, 1.000000000000000000, 0.000000000000000000 ) ) ;
#8191=VECTOR ( 'NONE', #16880, 1000.000000000000000 ) ;
#8193=AXIS2_PLACEMENT_3D ( 'NONE', #4312, #655, #768 ) ;
#8197=ORIENTED_EDGE ( 'NONE', *, *, #7376, .T. ) ;
#8218=CARTESIAN_POINT ( 'NONE',  ( -23.01875000000000071, 0.000000000000000000, -3.968750000000000000 ) ) ;
#8222=VECTOR ( 'NONE', #14086, 1000.000000000000000 ) ;
#8230=CARTESIAN_POINT ( 'NONE',  ( 0.02083138522552824973, 20.24316500000000119, 7.210477125664100484 ) ) ;
#8234=AXIS2_PLACEMENT_3D ( 'NONE', #10421, #8642, #1576 ) ;
#8249=ORIENTED_EDGE ( 'NONE', *, *, #15671, .T. ) ;
#8262=AXIS2_PLACEMENT_3D ( 'NONE', #9045, #15821, #17799 ) ;
#8264=CARTESIAN_POINT ( 'NONE',  ( 46.03750000000000142, 32.54502000000000095, -10.31874999999999964 ) ) ;
#8275=EDGE_LOOP ( 'NONE', ( #19321, #20165, #20811, #18234, #1709 ) ) ;
#8279=VECTOR ( 'NONE', #3151, 1000.000000000000000 ) ;
#8281=VERTEX_POINT ( 'NONE', #20550 ) ;
#8282=DIRECTION ( 'NONE',  ( 1.000000000000000000, 0.000000000000000000, 0.000000000000000000 ) ) ;
#8286=ADVANCED_FACE ( 'NONE', ( #5637 ), #20429, .F. ) ;
#8289=CARTESIAN_POINT ( 'NONE',  ( 70.64340948846358970, 1.984375000000000000, -10.53785647675949910 ) ) ;
#8302=CARTESIAN_POINT ( 'NONE',  ( 49.81956284419040060, 30.56064500000000095, 11.98436472153758103 ) ) ;
#8308=EDGE_CURVE ( 'NONE', #6054, #4933, #14068, .T. ) ;
#8311=CARTESIAN_POINT ( 'NONE',  ( 2.063749999518360134, 30.56070453124999986, 10.71562494997783865 ) ) ;
#8313=CARTESIAN_POINT ( 'NONE',  ( -2.607150795738780058, 32.54502000000000095, 8.731885000000000119 ) ) ;
#8322=EDGE_CURVE ( 'NONE', #12596, #10374, #8729, .T. ) ;
#8329=CARTESIAN_POINT ( 'NONE',  ( -29.36874999999999858, 1.984375000000000000, 8.731249999999999289 ) ) ;
#8343=LINE ( 'NONE', #18297, #13126 ) ;
#8360=VECTOR ( 'NONE', #14033, 1000.000000000000000 ) ;
#8364=CARTESIAN_POINT ( 'NONE',  ( 66.03921914090641110, 30.56064500000000095, -10.93409647675949969 ) ) ;
#8367=EDGE_CURVE ( 'NONE', #16212, #777, #12722, .T. ) ;
#8368=ORIENTED_EDGE ( 'NONE', *, *, #20284, .T. ) ;
#8372=DIRECTION ( 'NONE',  ( -0.9966381950048638361, 0.000000000000000000, 0.08192867786951606168 ) ) ;
#8376=VECTOR ( 'NONE', #5926, 1000.000000000000227 ) ;
#8378=ORIENTED_EDGE ( 'NONE', *, *, #6781, .F. ) ;
#8379=DIRECTION ( 'NONE',  ( 1.000000000000000000, 0.000000000000000000, 0.000000000000000000 ) ) ;
#8384=VECTOR ( 'NONE', #16165, 1000.000000000000000 ) ;
#8395=LINE ( 'NONE', #13302, #20900 ) ;
#8403=LINE ( 'NONE', #3553, #15844 ) ;
#8419=ORIENTED_EDGE ( 'NONE', *, *, #14543, .T. ) ;
#8428=ORIENTED_EDGE ( 'NONE', *, *, #9889, .F. ) ;
#8432=CARTESIAN_POINT ( 'NONE',  ( 65.90927232300019512, 1.984375000000000000, -13.30734117861468135 ) ) ;
#8433=AXIS2_PLACEMENT_3D ( 'NONE', #16890, #7045, #17332 ) ;
#8456=AXIS2_PLACEMENT_3D ( 'NONE', #19828, #16635, #6463 ) ;
#8461=AXIS2_PLACEMENT_3D ( 'NONE', #14083, #20910, #2340 ) ;
#8476=DIRECTION ( 'NONE',  ( -1.000000000000000000, 0.000000000000000000, 0.000000000000000000 ) ) ;
#8487=ORIENTED_EDGE ( 'NONE', *, *, #7490, .T. ) ;
#8488=ORIENTED_EDGE ( 'NONE', *, *, #5082, .T. ) ;
#8489=DIRECTION ( 'NONE',  ( 1.000000000000000000, 0.000000000000000000, 0.000000000000000000 ) ) ;
#8493=EDGE_CURVE ( 'NONE', #7268, #10232, #19337, .T. ) ;
#8494=CIRCLE ( 'NONE', #16643, 2.381250000000001421 ) ;
#8497=DIRECTION ( 'NONE',  ( 0.000000000000000000, -1.000000000000000000, 0.000000000000000000 ) ) ;
#8505=DIRECTION ( 'NONE',  ( -0.06191955310929833645, 0.000000000000000000, 0.9980811434661738257 ) ) ;
#8521=DIRECTION ( 'NONE',  ( 0.000000000000000000, -1.000000000000000000, 0.000000000000000000 ) ) ;
#8525=DIRECTION ( 'NONE',  ( 0.000000000000000000, 0.000000000000000000, -1.000000000000000000 ) ) ;
#8539=ORIENTED_EDGE ( 'NONE', *, *, #9567, .F. ) ;
#8544=ORIENTED_EDGE ( 'NONE', *, *, #7769, .T. ) ;
#8561=LINE ( 'NONE', #3384, #13441 ) ;
#8568=DIRECTION ( 'NONE',  ( 0.000000000000000000, 1.000000000000000000, 0.000000000000000000 ) ) ;
#8569=CARTESIAN_POINT ( 'NONE',  ( 70.64340948846358970, 1.984375000000000000, -10.93409647675949969 ) ) ;
#8575=CARTESIAN_POINT ( 'NONE',  ( 1.268730000000000135, 23.41816500000000190, 10.65596716962832069 ) ) ;
#8580=DIRECTION ( 'NONE',  ( 1.000000000000000000, 0.000000000000000000, 0.000000000000000000 ) ) ;
#8581=EDGE_LOOP ( 'NONE', ( #21875, #9659, #16668, #5526 ) ) ;
#8589=VERTEX_POINT ( 'NONE', #1859 ) ;
#8603=ORIENTED_EDGE ( 'NONE', *, *, #15751, .F. ) ;
#8605=CARTESIAN_POINT ( 'NONE',  ( 1.268730000000000135, 24.21318500000000284, 10.71562499999999929 ) ) ;
#8610=ORIENTED_EDGE ( 'NONE', *, *, #4694, .T. ) ;
#8613=DIRECTION ( 'NONE',  ( -0.1831666983862943188, 0.000000000000000000, 0.9830818687180962190 ) ) ;
#8634=DIRECTION ( 'NONE',  ( 0.000000000000000000, 1.000000000000000000, 0.000000000000000000 ) ) ;
#8636=LINE ( 'NONE', #16826, #5056 ) ;
#8640=FACE_OUTER_BOUND ( 'NONE', #206, .T. ) ;
#8642=DIRECTION ( 'NONE',  ( 1.000000000000000000, 0.000000000000000000, 0.000000000000000000 ) ) ;
#8651=VERTEX_POINT ( 'NONE', #20637 ) ;
#8655=CARTESIAN_POINT ( 'NONE',  ( 49.81956284419040060, 30.56064500000000095, 11.98436472153758103 ) ) ;
#8659=DIRECTION ( 'NONE',  ( 0.000000000000000000, 1.000000000000000000, 0.000000000000000000 ) ) ;
#8675=ORIENTED_EDGE ( 'NONE', *, *, #21417, .F. ) ;
#8683=ORIENTED_EDGE ( 'NONE', *, *, #10600, .F. ) ;
#8684=DIRECTION ( 'NONE',  ( 0.000000000000000000, 0.000000000000000000, -1.000000000000000000 ) ) ;
#8685=ORIENTED_EDGE ( 'NONE', *, *, #20965, .F. ) ;
#8691=DIRECTION ( 'NONE',  ( 0.000000000000000000, -1.000000000000000000, 0.000000000000000000 ) ) ;
#8712=ORIENTED_EDGE ( 'NONE', *, *, #3615, .T. ) ;
#8725=DIRECTION ( 'NONE',  ( 0.000000000000000000, 1.000000000000000000, 0.000000000000000000 ) ) ;
#8729=LINE ( 'NONE', #17032, #19815 ) ;
#8731=ORIENTED_EDGE ( 'NONE', *, *, #6622, .F. ) ;
#8736=DIRECTION ( 'NONE',  ( 0.000000000000000000, 0.000000000000000000, -1.000000000000000000 ) ) ;
#8744=DIRECTION ( 'NONE',  ( 0.000000000000000000, 0.000000000000000000, -1.000000000000000000 ) ) ;
#8747=CARTESIAN_POINT ( 'NONE',  ( 26.59062499999999929, 26.59189500000000095, 10.71562499999999929 ) ) ;
#8759=FACE_OUTER_BOUND ( 'NONE', #13153, .T. ) ;
#8762=AXIS2_PLACEMENT_3D ( 'NONE', #1655, #21785, #13397 ) ;
#8773=VERTEX_POINT ( 'NONE', #9138 ) ;
#8778=CIRCLE ( 'NONE', #1728, 25.00312500000000426 ) ;
#8785=CARTESIAN_POINT ( 'NONE',  ( 24.60624999999999929, 16.27314499999999953, 10.71562499999999929 ) ) ;
#8786=ORIENTED_EDGE ( 'NONE', *, *, #9786, .T. ) ;
#8790=EDGE_LOOP ( 'NONE', ( #16139, #9695, #4343, #17303, #10726, #8197, #417, #154, #21571, #9958, #1076, #1931 ) ) ;
#8796=LINE ( 'NONE', #12142, #8360 ) ;
#8801=DIRECTION ( 'NONE',  ( 0.000000000000000000, 0.000000000000000000, 1.000000000000000000 ) ) ;
#8805=VERTEX_POINT ( 'NONE', #2412 ) ;
#8819=EDGE_CURVE ( 'NONE', #18667, #11600, #19095, .T. ) ;
#8825=DIRECTION ( 'NONE',  ( 0.9876802608827758290, 0.000000000000000000, -0.1564854698127972066 ) ) ;
#8828=FACE_BOUND ( 'NONE', #4018, .T. ) ;
#8838=VECTOR ( 'NONE', #2034, 1000.000000000000000 ) ;
#8849=VECTOR ( 'NONE', #8170, 1000.000000000000000 ) ;
#8863=CIRCLE ( 'NONE', #5328, 0.3962399999999997591 ) ;
#8868=ADVANCED_FACE ( 'NONE', ( #21300 ), #7497, .F. ) ;
#8871=CARTESIAN_POINT ( 'NONE',  ( 49.41235866845560309, 0.000000000000000000, -26.78690084448080100 ) ) ;
#8873=AXIS2_PLACEMENT_3D ( 'NONE', #19791, #20296, #11916 ) ;
#8876=FACE_OUTER_BOUND ( 'NONE', #7739, .T. ) ;
#8879=VECTOR ( 'NONE', #14968, 1000.000000000000000 ) ;
#8891=ORIENTED_EDGE ( 'NONE', *, *, #14396, .T. ) ;
#8910=ORIENTED_EDGE ( 'NONE', *, *, #21706, .F. ) ;
#8922=DIRECTION ( 'NONE',  ( 0.000000000000000000, 0.000000000000000000, -1.000000000000000000 ) ) ;
#8945=PLANE ( 'NONE',  #13361 ) ;
#8954=EDGE_CURVE ( 'NONE', #13795, #15382, #10259, .T. ) ;
#8955=EDGE_CURVE ( 'NONE', #2722, #10050, #21408, .T. ) ;
#8959=EDGE_LOOP ( 'NONE', ( #2167, #3613 ) ) ;
#8972=DIRECTION ( 'NONE',  ( -0.9579671649362032637, 0.000000000000000000, 0.2868778675745010664 ) ) ;
#8979=EDGE_CURVE ( 'NONE', #14819, #12179, #14704, .T. ) ;
#8994=ADVANCED_FACE ( 'NONE', ( #16665 ), #11680, .F. ) ;
#8997=EDGE_CURVE ( 'NONE', #3294, #6310, #4613, .T. ) ;
#9002=CARTESIAN_POINT ( 'NONE',  ( -29.36874999999999858, 30.56064500000000095, -3.968750000000000000 ) ) ;
#9016=VERTEX_POINT ( 'NONE', #1394 ) ;
#9022=AXIS2_PLACEMENT_3D ( 'NONE', #18067, #20025, #8096 ) ;
#9027=EDGE_LOOP ( 'NONE', ( #1882, #14028, #12561, #19160 ) ) ;
#9031=VERTEX_POINT ( 'NONE', #16457 ) ;
#9032=EDGE_LOOP ( 'NONE', ( #20292, #5902, #15868, #4321 ) ) ;
#9038=EDGE_LOOP ( 'NONE', ( #19638, #9836, #19493, #19851 ) ) ;
#9042=ADVANCED_FACE ( 'NONE', ( #20172 ), #2965, .T. ) ;
#9043=CARTESIAN_POINT ( 'NONE',  ( -2.607150795738780058, 0.000000000000000000, 8.731885000000000119 ) ) ;
#9045=CARTESIAN_POINT ( 'NONE',  ( 21.43124999999999858, 16.27314499999999953, 10.71562499999999929 ) ) ;
#9052=CARTESIAN_POINT ( 'NONE',  ( -1.000942312354703878, 9.129395000000000593, 10.71562499999999929 ) ) ;
#9081=CARTESIAN_POINT ( 'NONE',  ( 151.3494547525804990, 22.62314500000000095, -45.56305690039940259 ) ) ;
#9086=VECTOR ( 'NONE', #442, 1000.000000000000227 ) ;
#9088=LINE ( 'NONE', #17945, #21138 ) ;
#9103=LINE ( 'NONE', #9002, #2122 ) ;
#9117=CARTESIAN_POINT ( 'NONE',  ( 2.063750000000000195, 30.16440499999999858, 8.731249999999999289 ) ) ;
#9118=ADVANCED_FACE ( 'NONE', ( #20612 ), #15681, .F. ) ;
#9126=EDGE_LOOP ( 'NONE', ( #11341, #14645 ) ) ;
#9131=CIRCLE ( 'NONE', #21856, 3.968750000000000000 ) ;
#9132=EDGE_LOOP ( 'NONE', ( #2736, #8544 ) ) ;
#9134=CARTESIAN_POINT ( 'NONE',  ( 0.02083138522551555155, 12.30439499999999953, 7.210477125664100484 ) ) ;
#9138=CARTESIAN_POINT ( 'NONE',  ( 2.063750000000000195, 8.334374999999999645, 8.731249999999999289 ) ) ;
#9142=VERTEX_POINT ( 'NONE', #18628 ) ;
#9145=VECTOR ( 'NONE', #14119, 1000.000000000000000 ) ;
#9148=CIRCLE ( 'NONE', #8456, 0.3962400000000008138 ) ;
#9151=CARTESIAN_POINT ( 'NONE',  ( 5.447351731530780228, 1.984375000000000000, 0.8930339070797439494 ) ) ;
#9156=DIRECTION ( 'NONE',  ( 0.000000000000000000, 0.000000000000000000, 1.000000000000000000 ) ) ;
#9157=CARTESIAN_POINT ( 'NONE',  ( 54.11611804786240043, 0.000000000000000000, -30.58983753981140197 ) ) ;
#9162=LINE ( 'NONE', #4318, #17895 ) ;
#9168=CARTESIAN_POINT ( 'NONE',  ( 66.03921914090641110, 30.56064500000000095, -10.93409647675949969 ) ) ;
#9173=CIRCLE ( 'NONE', #11993, 25.00312500000000426 ) ;
#9178=DIRECTION ( 'NONE',  ( -0.5733392046337749681, 0.8193181045417647912, 0.000000000000000000 ) ) ;
#9184=CARTESIAN_POINT ( 'NONE',  ( 67.40134256979101224, 74.97070807199999365, -13.70358117861468017 ) ) ;
#9189=VERTEX_POINT ( 'NONE', #13790 ) ;
#9202=DIRECTION ( 'NONE',  ( 0.000000000000000000, -1.000000000000000000, 0.000000000000000000 ) ) ;
#9205=ORIENTED_EDGE ( 'NONE', *, *, #15319, .T. ) ;
#9218=VECTOR ( 'NONE', #10970, 1000.000000000000227 ) ;
#9234=ORIENTED_EDGE ( 'NONE', *, *, #15634, .T. ) ;
#9237=ORIENTED_EDGE ( 'NONE', *, *, #18721, .T. ) ;
#9238=CYLINDRICAL_SURFACE ( 'NONE', #20557, 19.05000000000000426 ) ;
#9240=EDGE_CURVE ( 'NONE', #14134, #19333, #20480, .T. ) ;
#9242=VECTOR ( 'NONE', #4634, 1000.000000000000000 ) ;
#9247=ORIENTED_EDGE ( 'NONE', *, *, #5374, .F. ) ;
#9249=AXIS2_PLACEMENT_3D ( 'NONE', #18468, #17027, #8505 ) ;
#9262=DIRECTION ( 'NONE',  ( 0.000000000000000000, 1.000000000000000000, 0.000000000000000000 ) ) ;
#9279=CARTESIAN_POINT ( 'NONE',  ( 26.59062499999999929, 30.16440499999999858, 8.731249999999999289 ) ) ;
#9292=CIRCLE ( 'NONE', #21655, 0.3962400000000008138 ) ;
#9295=ADVANCED_BREP_SHAPE_REPRESENTATION ( '', ( #6635, #2234 ), #16895 ) ;
#9304=CARTESIAN_POINT ( 'NONE',  ( 1.954387715434429795, 23.81077936178774834, 10.71562499999999929 ) ) ;
#9305=DIRECTION ( 'NONE',  ( 0.9579671649362033747, 0.000000000000000000, -0.2868778675745011220 ) ) ;
#9316=PLANE ( 'NONE',  #12772 ) ;
#9320=AXIS2_PLACEMENT_3D ( 'NONE', #19995, #16708, #12048 ) ;
#9321=ORIENTED_EDGE ( 'NONE', *, *, #10902, .T. ) ;
#9326=DIRECTION ( 'NONE',  ( 1.000000000000000000, 0.000000000000000000, 0.000000000000000000 ) ) ;
#9328=CARTESIAN_POINT ( 'NONE',  ( -23.01875000000000071, 30.56064500000000095, -10.31874999999999964 ) ) ;
#9335=EDGE_LOOP ( 'NONE', ( #20889, #505, #5035, #14593 ) ) ;
#9360=EDGE_LOOP ( 'NONE', ( #12841, #16340, #15120, #6399 ) ) ;
#9373=EDGE_CURVE ( 'NONE', #15989, #3518, #16219, .T. ) ;
#9396=CARTESIAN_POINT ( 'NONE',  ( 55.56250000000000000, 0.000000000000000000, -10.31874999999999964 ) ) ;
#9413=CARTESIAN_POINT ( 'NONE',  ( -29.36874999999999858, 1.984375000000000000, -13.26881841860929967 ) ) ;
#9426=ADVANCED_FACE ( 'NONE', ( #19183 ), #14241, .F. ) ;
#9430=DIRECTION ( 'NONE',  ( 0.000000000000000000, 0.000000000000000000, -1.000000000000000000 ) ) ;
#9433=DIRECTION ( 'NONE',  ( -0.6287118719681975554, 0.000000000000000000, -0.7776383362760898033 ) ) ;
#9438=EDGE_LOOP ( 'NONE', ( #12054, #21067, #6350, #5614 ) ) ;
#9441=EDGE_LOOP ( 'NONE', ( #15094, #4916, #12608, #11004 ) ) ;
#9449=FACE_OUTER_BOUND ( 'NONE', #8139, .T. ) ;
#9456=VERTEX_POINT ( 'NONE', #12672 ) ;
#9462=VERTEX_POINT ( 'NONE', #19394 ) ;
#9471=DIRECTION ( 'NONE',  ( 1.000000000000000000, 0.000000000000000000, 0.000000000000000000 ) ) ;
#9476=ORIENTED_EDGE ( 'NONE', *, *, #17962, .T. ) ;
#9491=VECTOR ( 'NONE', #20630, 1000.000000000000000 ) ;
#9519=ORIENTED_EDGE ( 'NONE', *, *, #6603, .T. ) ;
#9532=CARTESIAN_POINT ( 'NONE',  ( 6.585898268469219552, 1.984375000000000000, 4.694966092919240275 ) ) ;
#9533=VECTOR ( 'NONE', #17376, 1000.000000000000000 ) ;
#9541=DIRECTION ( 'NONE',  ( 0.000000000000000000, -1.000000000000000000, 0.000000000000000000 ) ) ;
#9543=EDGE_CURVE ( 'NONE', #1202, #15261, #19458, .T. ) ;
#9545=FACE_OUTER_BOUND ( 'NONE', #2694, .T. ) ;
#9546=VECTOR ( 'NONE', #5078, 1000.000000000000000 ) ;
#9547=VERTEX_POINT ( 'NONE', #1593 ) ;
#9550=ORIENTED_EDGE ( 'NONE', *, *, #4239, .F. ) ;
#9567=EDGE_CURVE ( 'NONE', #2328, #18667, #20035, .T. ) ;
#9568=CARTESIAN_POINT ( 'NONE',  ( 66.03921914090641110, -42.42568807200000691, -11.33033647675950029 ) ) ;
#9571=DIRECTION ( 'NONE',  ( 0.000000000000000000, 1.000000000000000000, 0.000000000000000000 ) ) ;
#9606=CARTESIAN_POINT ( 'NONE',  ( -29.36874999999999858, 32.54502000000000095, -3.968750000000000000 ) ) ;
#9619=CARTESIAN_POINT ( 'NONE',  ( 21.03437500000000071, 1.984375000000000000, 5.159374999999999822 ) ) ;
#9623=EDGE_CURVE ( 'NONE', #15261, #7667, #8863, .T. ) ;
#9625=EDGE_CURVE ( 'NONE', #5674, #7354, #14544, .T. ) ;
#9626=EDGE_LOOP ( 'NONE', ( #3576, #2415, #1182, #14467 ) ) ;
#9629=DIRECTION ( 'NONE',  ( 0.9876802608827758290, 0.000000000000000000, -0.1564854698127972066 ) ) ;
#9632=DIRECTION ( 'NONE',  ( 0.000000000000000000, 1.000000000000000000, 0.000000000000000000 ) ) ;
#9634=AXIS2_PLACEMENT_3D ( 'NONE', #1895, #8525, #17048 ) ;
#9636=ORIENTED_EDGE ( 'NONE', *, *, #15908, .T. ) ;
#9649=CARTESIAN_POINT ( 'NONE',  ( 23.41562500000000213, 30.56064500000000095, 5.159374999999999822 ) ) ;
#9659=ORIENTED_EDGE ( 'NONE', *, *, #943, .F. ) ;
#9666=ORIENTED_EDGE ( 'NONE', *, *, #18993, .T. ) ;
#9669=ORIENTED_EDGE ( 'NONE', *, *, #14654, .T. ) ;
#9678=CARTESIAN_POINT ( 'NONE',  ( -23.01875000000000071, 0.000000000000000000, -10.31874999999999964 ) ) ;
#9684=DIRECTION ( 'NONE',  ( 0.000000000000000000, -1.000000000000000000, 0.000000000000000000 ) ) ;
#9687=VERTEX_POINT ( 'NONE', #8655 ) ;
#9691=CARTESIAN_POINT ( 'NONE',  ( -160.2647810241784896, 30.56128000000000000, 8.731885000000000119 ) ) ;
#9695=ORIENTED_EDGE ( 'NONE', *, *, #11173, .T. ) ;
#9698=EDGE_CURVE ( 'NONE', #19545, #16113, #16600, .T. ) ;
#9700=CIRCLE ( 'NONE', #10787, 3.175000000000000711 ) ;
#9709=LINE ( 'NONE', #1307, #9242 ) ;
#9711=CARTESIAN_POINT ( 'NONE',  ( 18.65312499999999929, 32.54502000000000095, 5.159374999999999822 ) ) ;
#9712=B_SPLINE_CURVE_WITH_KNOTS ( 'NONE', 3,
 ( #6932, #20510, #2055, #17444, #2173, #13695, #3843, #18640 ),
 .UNSPECIFIED., .F., .F.,
 ( 4, 2, 2, 4 ),
 ( 0.000000000000000000, 0.2500000000000000000, 0.5000000000000000000, 1.000000000000000000 ),
 .UNSPECIFIED. ) ;
#9718=ORIENTED_EDGE ( 'NONE', *, *, #1432, .F. ) ;
#9721=LINE ( 'NONE', #4862, #18028 ) ;
#9731=DIRECTION ( 'NONE',  ( 0.000000000000000000, -1.000000000000000000, 0.000000000000000000 ) ) ;
#9738=FACE_OUTER_BOUND ( 'NONE', #6963, .T. ) ;
#9745=DIRECTION ( 'NONE',  ( 0.000000000000000000, 0.000000000000000000, 1.000000000000000000 ) ) ;
#9746=ADVANCED_FACE ( 'NONE', ( #6670 ), #17064, .T. ) ;
#9748=DIRECTION ( 'NONE',  ( -0.6287118719681937806, 0.000000000000000000, -0.7776383362760928009 ) ) ;
#9765=DIRECTION ( 'NONE',  ( -1.000000000000000000, 0.000000000000000000, 0.000000000000000000 ) ) ;
#9767=DIRECTION ( 'NONE',  ( 0.000000000000000000, 1.000000000000000000, 0.000000000000000000 ) ) ;
#9772=CARTESIAN_POINT ( 'NONE',  ( 66.87634738983680904, 1.984375000000000000, 3.497859541731999755 ) ) ;
#9776=CARTESIAN_POINT ( 'NONE',  ( 201.9384738932629944, 1.984375000000000000, 10.71562489836746046 ) ) ;
#9786=EDGE_CURVE ( 'NONE', #3005, #21819, #13780, .T. ) ;
#9792=CYLINDRICAL_SURFACE ( 'NONE', #14133, 3.968750000000000000 ) ;
#9795=VERTEX_POINT ( 'NONE', #16949 ) ;
#9797=EDGE_LOOP ( 'NONE', ( #18313, #19205, #11212, #6189 ) ) ;
#9799=ORIENTED_EDGE ( 'NONE', *, *, #5708, .F. ) ;
#9800=DIRECTION ( 'NONE',  ( 0.000000000000000000, 1.000000000000000000, 0.000000000000000000 ) ) ;
#9801=ORIENTED_EDGE ( 'NONE', *, *, #896, .F. ) ;
#9809=VERTEX_POINT ( 'NONE', #7969 ) ;
#9812=CARTESIAN_POINT ( 'NONE',  ( 54.36523883999320361, 32.54502000000000095, -30.28170612544299800 ) ) ;
#9815=ORIENTED_EDGE ( 'NONE', *, *, #4129, .F. ) ;
#9825=CIRCLE ( 'NONE', #3859, 0.3962400000000008138 ) ;
#9833=DIRECTION ( 'NONE',  ( 1.000000000000000000, 0.000000000000000000, 0.000000000000000000 ) ) ;
#9836=ORIENTED_EDGE ( 'NONE', *, *, #17897, .T. ) ;
#9850=DIRECTION ( 'NONE',  ( 0.000000000000000000, 1.000000000000000000, 0.000000000000000000 ) ) ;
#9854=CIRCLE ( 'NONE', #13416, 3.968750000000000000 ) ;
#9856=LINE ( 'NONE', #18489, #3382 ) ;
#9858=AXIS2_PLACEMENT_3D ( 'NONE', #2591, #6001, #1346 ) ;
#9859=CARTESIAN_POINT ( 'NONE',  ( 26.59062499999999929, 26.59189500000000095, 8.731249999999999289 ) ) ;
#9860=ADVANCED_FACE ( 'NONE', ( #19784 ), #16809, .T. ) ;
#9870=DIRECTION ( 'NONE',  ( 0.000000000000000000, 1.000000000000000000, 0.000000000000000000 ) ) ;
#9872=PLANE ( 'NONE',  #6389 ) ;
#9876=CARTESIAN_POINT ( 'NONE',  ( 31.75000000000000000, 1.984375000000000000, -4.317999999999999616 ) ) ;
#9886=FACE_OUTER_BOUND ( 'NONE', #664, .T. ) ;
#9889=EDGE_CURVE ( 'NONE', #12065, #14993, #21807, .T. ) ;
#9894=LINE ( 'NONE', #4927, #19105 ) ;
#9896=ORIENTED_EDGE ( 'NONE', *, *, #14904, .F. ) ;
#9899=DIRECTION ( 'NONE',  ( 0.000000000000000000, 0.000000000000000000, 1.000000000000000000 ) ) ;
#9910=ADVANCED_FACE ( 'NONE', ( #4770 ), #18150, .F. ) ;
#9913=FACE_OUTER_BOUND ( 'NONE', #19597, .T. ) ;
#9915=VECTOR ( 'NONE', #13345, 1000.000000000000000 ) ;
#9916=FACE_OUTER_BOUND ( 'NONE', #7342, .T. ) ;
#9919=AXIS2_PLACEMENT_3D ( 'NONE', #6470, #4486, #4591 ) ;
#9921=EDGE_CURVE ( 'NONE', #10689, #18275, #13187, .T. ) ;
#9923=CARTESIAN_POINT ( 'NONE',  ( 70.64340948846358970, 32.54502000000000095, -10.53785647675949910 ) ) ;
#9933=EDGE_LOOP ( 'NONE', ( #17767, #21158, #12181, #7028 ) ) ;
#9939=CLOSED_SHELL ( 'NONE', ( #12314, #5130, #7289, #1659, #3174, #9118, #8286, #20285, #11694, #11427, #13760, #11105, #16019, #7338, #14895, #1385, #13612, #4395, #16804, #18856, #7266, #4247, #14005, #9860, #6322, #4350, #8994, #20983, #6542, #5085, #10806, #743, #6762, #18724, #15647, #13689, #13272, #8868, #4885, #1975, #14269, #15353, #17120, #13297, #3711, #1386, #15744, #6582, #3839, #2344, #19589, #18954, #4950, #1168, #10782, #2228, #19077, #11577, #21089, #6256, #9746, #7562, #9042, #9426, #14683, #16652, #5683, #7639, #9, #2343, #13738, #20157, #13121, #5767, #4764, #10448, #11929, #3819, #16598, #16415, #3323, #17116, #14973, #17373, #12736, #7607, #3074, #18577, #17477, #9910, #4514, #16779, #16407, #8122, #5063, #17523, #13221, #10073, #16307, #922, #15416, #5972 ) ) ;
#9947=CARTESIAN_POINT ( 'NONE',  ( 28.97711086133420366, 0.000000000000000000, -10.31874999999999964 ) ) ;
#9953=CARTESIAN_POINT ( 'NONE',  ( 2.063750000000000195, 2.380615000000000148, 8.731249999999999289 ) ) ;
#9954=LINE ( 'NONE', #16715, #7823 ) ;
#9958=ORIENTED_EDGE ( 'NONE', *, *, #13537, .F. ) ;
#9963=ORIENTED_EDGE ( 'NONE', *, *, #7265, .T. ) ;
#9966=CIRCLE ( 'NONE', #19856, 0.3962400000000008138 ) ;
#9971=ORIENTED_EDGE ( 'NONE', *, *, #12382, .F. ) ;
#9991=ORIENTED_EDGE ( 'NONE', *, *, #10605, .T. ) ;
#9994=CYLINDRICAL_SURFACE ( 'NONE', #17036, 6.349999999999997868 ) ;
#10019=ORIENTED_EDGE ( 'NONE', *, *, #9698, .F. ) ;
#10026=ORIENTED_EDGE ( 'NONE', *, *, #5863, .F. ) ;
#10027=ORIENTED_EDGE ( 'NONE', *, *, #17287, .F. ) ;
#10046=EDGE_LOOP ( 'NONE', ( #11495, #5090, #10969, #10123, #1421 ) ) ;
#10049=VECTOR ( 'NONE', #14325, 1000.000000000000227 ) ;
#10050=VERTEX_POINT ( 'NONE', #17022 ) ;
#10053=CARTESIAN_POINT ( 'NONE',  ( -160.2647810241784896, 30.16440499999999858, 8.335010000000000474 ) ) ;
#10056=EDGE_CURVE ( 'NONE', #8805, #10374, #20316, .T. ) ;
#10073=ADVANCED_FACE ( 'NONE', ( #8828, #13617, #7194, #13835, #1756 ), #8945, .T. ) ;
#10074=EDGE_CURVE ( 'NONE', #9031, #16780, #2087, .T. ) ;
#10086=DIRECTION ( 'NONE',  ( 0.000000000000000000, -1.000000000000000000, 0.000000000000000000 ) ) ;
#10099=DIRECTION ( 'NONE',  ( 0.000000000000000000, 1.000000000000000000, 0.000000000000000000 ) ) ;
#10115=PRODUCT_DEFINITION_CONTEXT ( 'detailed design', #20907, 'design' ) ;
#10123=ORIENTED_EDGE ( 'NONE', *, *, #5107, .F. ) ;
#10133=CARTESIAN_POINT ( 'NONE',  ( 29.36887348155339694, 30.56064500123875050, 10.71562877576799977 ) ) ;
#10141=CARTESIAN_POINT ( 'NONE',  ( 30.33489826846160398, 1.984375000000000000, -2.417033907079745525 ) ) ;
#10144=DIRECTION ( 'NONE',  ( 0.000000000000000000, -1.000000000000000000, 0.000000000000000000 ) ) ;
#10154=CARTESIAN_POINT ( 'NONE',  ( -1.345424459097947834, 12.30439499999999953, 2.648158502653860324 ) ) ;
#10158=VECTOR ( 'NONE', #16063, 1000.000000000000000 ) ;
#10162=CARTESIAN_POINT ( 'NONE',  ( 65.90927232300019512, -42.42568807200000691, -12.91110117861467899 ) ) ;
#10164=CARTESIAN_POINT ( 'NONE',  ( -1.848761088705630051, 23.41816500000000190, 7.884515871828260636 ) ) ;
#10172=EDGE_CURVE ( 'NONE', #2822, #6097, #20976, .T. ) ;
#10174=EDGE_CURVE ( 'NONE', #19683, #21868, #14150, .T. ) ;
#10186=CYLINDRICAL_SURFACE ( 'NONE', #6704, 9.524999999999998579 ) ;
#10189=AXIS2_PLACEMENT_3D ( 'NONE', #21654, #12950, #21759 ) ;
#10197=EDGE_CURVE ( 'NONE', #4510, #6097, #21075, .T. ) ;
#10205=CARTESIAN_POINT ( 'NONE',  ( 29.36874999999999858, 0.000000000000000000, 10.71562499999999929 ) ) ;
#10215=EDGE_CURVE ( 'NONE', #6097, #19275, #19414, .T. ) ;
#10222=ORIENTED_EDGE ( 'NONE', *, *, #6622, .T. ) ;
#10231=DIRECTION ( 'NONE',  ( 3.502369222646484109E-14, 0.000000000000000000, 1.000000000000000000 ) ) ;
#10232=VERTEX_POINT ( 'NONE', #7703 ) ;
#10234=AXIS2_PLACEMENT_3D ( 'NONE', #290, #2370, #7031 ) ;
#10240=EDGE_CURVE ( 'NONE', #2714, #18576, #19203, .T. ) ;
#10247=CARTESIAN_POINT ( 'NONE',  ( 54.36523883999320361, 30.56064500000000095, -30.28170612544299800 ) ) ;
#10251=FACE_BOUND ( 'NONE', #2465, .T. ) ;
#10259=CIRCLE ( 'NONE', #13111, 0.3962400000000008138 ) ;
#10267=EDGE_CURVE ( 'NONE', #9142, #9809, #738, .T. ) ;
#10269=AXIS2_PLACEMENT_3D ( 'NONE', #14681, #6241, #13014 ) ;
#10273=DIRECTION ( 'NONE',  ( 0.000000000000000000, 0.000000000000000000, 1.000000000000000000 ) ) ;
#10274=ORIENTED_EDGE ( 'NONE', *, *, #2620, .T. ) ;
#10284=ORIENTED_EDGE ( 'NONE', *, *, #10498, .F. ) ;
#10285=CIRCLE ( 'NONE', #3586, 22.02656249999999005 ) ;
#10287=CIRCLE ( 'NONE', #11719, 0.3962399999999975386 ) ;
#10293=DIRECTION ( 'NONE',  ( 0.000000000000000000, -1.000000000000000000, 0.000000000000000000 ) ) ;
#10295=VECTOR ( 'NONE', #2866, 1000.000000000000000 ) ;
#10301=EDGE_CURVE ( 'NONE', #11142, #14819, #14360, .T. ) ;
#10302=AXIS2_PLACEMENT_3D ( 'NONE', #8264, #13691, #20076 ) ;
#10305=VECTOR ( 'NONE', #18329, 1000.000000000000000 ) ;
#10309=CARTESIAN_POINT ( 'NONE',  ( 29.37324403177899868, 32.54502000000000095, -10.70578951775076071 ) ) ;
#10320=VERTEX_POINT ( 'NONE', #5603 ) ;
#10353=FACE_OUTER_BOUND ( 'NONE', #564, .T. ) ;
#10354=EDGE_CURVE ( 'NONE', #8651, #21849, #7346, .T. ) ;
#10355=ORIENTED_EDGE ( 'NONE', *, *, #7883, .T. ) ;
#10362=CARTESIAN_POINT ( 'NONE',  ( -0.6285274567219200081, 1.984375000000000000, 8.854636014509949860 ) ) ;
#10370=DIRECTION ( 'NONE',  ( -0.000000000000000000, 1.000000000000000000, 0.000000000000000000 ) ) ;
#10374=VERTEX_POINT ( 'NONE', #11746 ) ;
#10379=ORIENTED_EDGE ( 'NONE', *, *, #10430, .F. ) ;
#10386=AXIS2_PLACEMENT_3D ( 'NONE', #18889, #648, #8825 ) ;
#10389=VECTOR ( 'NONE', #7134, 1000.000000000000000 ) ;
#10401=EDGE_LOOP ( 'NONE', ( #5759, #8038 ) ) ;
#10415=FACE_OUTER_BOUND ( 'NONE', #9360, .T. ) ;
#10421=CARTESIAN_POINT ( 'NONE',  ( -29.36874999999999858, 30.16440499999999858, 8.335010000000000474 ) ) ;
#10428=DIRECTION ( 'NONE',  ( 1.000000000000000000, 0.000000000000000000, 0.000000000000000000 ) ) ;
#10430=EDGE_CURVE ( 'NONE', #17367, #4043, #15512, .T. ) ;
#10435=DIRECTION ( 'NONE',  ( 0.000000000000000000, 1.000000000000000000, 0.000000000000000000 ) ) ;
#10438=VECTOR ( 'NONE', #2929, 1000.000000000000000 ) ;
#10440=CARTESIAN_POINT ( 'NONE',  ( 71.04062499999999147, 0.000000000000000000, -10.31874999999999964 ) ) ;
#10448=ADVANCED_FACE ( 'NONE', ( #13406 ), #5306, .T. ) ;
#10473=DIRECTION ( 'NONE',  ( 1.000000000000000000, 0.000000000000000000, 0.000000000000000000 ) ) ;
#10476=CARTESIAN_POINT ( 'NONE',  ( 67.79270099634359781, 32.54502000000000095, -13.76558698117381851 ) ) ;
#10477=CARTESIAN_POINT ( 'NONE',  ( 5.447351731530780228, 0.000000000000000000, 0.8930339070797439494 ) ) ;
#10487=ORIENTED_EDGE ( 'NONE', *, *, #6375, .T. ) ;
#10495=CARTESIAN_POINT ( 'NONE',  ( 1.597882609860227454, 23.48611691159180381, 8.700201306427871373 ) ) ;
#10498=EDGE_CURVE ( 'NONE', #10232, #12825, #8403, .T. ) ;
#10500=VECTOR ( 'NONE', #7806, 1000.000000000000000 ) ;
#10510=ORIENTED_EDGE ( 'NONE', *, *, #979, .F. ) ;
#10514=CARTESIAN_POINT ( 'NONE',  ( 18.65312499999999929, 32.54502000000000095, 5.159374999999999822 ) ) ;
#10524=CARTESIAN_POINT ( 'NONE',  ( 67.79270099634359781, 0.000000000000000000, -13.76558698117381851 ) ) ;
#10547=DIRECTION ( 'NONE',  ( 0.000000000000000000, -1.000000000000000000, 0.000000000000000000 ) ) ;
#10550=VECTOR ( 'NONE', #11093, 1000.000000000000000 ) ;
#10559=AXIS2_PLACEMENT_3D ( 'NONE', #5951, #4428, #12508 ) ;
#10569=FACE_OUTER_BOUND ( 'NONE', #8145, .T. ) ;
#10572=AXIS2_PLACEMENT_3D ( 'NONE', #18476, #16405, #11419 ) ;
#10574=ORIENTED_EDGE ( 'NONE', *, *, #14699, .F. ) ;
#10586=AXIS2_PLACEMENT_3D ( 'NONE', #3645, #7064, #2079 ) ;
#10600=EDGE_CURVE ( 'NONE', #14925, #18990, #20559, .T. ) ;
#10605=EDGE_CURVE ( 'NONE', #20984, #11600, #13974, .T. ) ;
#10625=CARTESIAN_POINT ( 'NONE',  ( 49.81956284419040060, 0.000000000000000000, 11.98436472153758103 ) ) ;
#10629=EDGE_CURVE ( 'NONE', #218, #16113, #19244, .T. ) ;
#10633=VECTOR ( 'NONE', #13461, 1000.000000000000000 ) ;
#10643=LINE ( 'NONE', #5873, #5298 ) ;
#10646=DIRECTION ( 'NONE',  ( -0.9579671649362034858, 0.000000000000000000, 0.2868778675745011220 ) ) ;
#10648=DIRECTION ( 'NONE',  ( 1.000000000000000000, 0.000000000000000000, 0.000000000000000000 ) ) ;
#10656=EDGE_LOOP ( 'NONE', ( #15656, #17616 ) ) ;
#10657=PRODUCT_CONTEXT ( 'NONE', #12720, 'mechanical' ) ;
#10658=DIRECTION ( 'NONE',  ( 1.000000000000000000, 0.000000000000000000, 0.000000000000000000 ) ) ;
#10662=VECTOR ( 'NONE', #17502, 1000.000000000000000 ) ;
#10679=ORIENTED_EDGE ( 'NONE', *, *, #12848, .T. ) ;
#10680=CIRCLE ( 'NONE', #18377, 3.175000000000000711 ) ;
#10689=VERTEX_POINT ( 'NONE', #5645 ) ;
#10695=AXIS2_PLACEMENT_3D ( 'NONE', #17323, #19080, #7485 ) ;
#10699=CIRCLE ( 'NONE', #16357, 3.970019999999998550 ) ;
#10703=DIRECTION ( 'NONE',  ( 0.000000000000000000, -1.000000000000000000, 0.000000000000000000 ) ) ;
#10719=ORIENTED_EDGE ( 'NONE', *, *, #641, .F. ) ;
#10723=CARTESIAN_POINT ( 'NONE',  ( -3.246390552019219999, 12.30439499999999953, 3.217431771123079987 ) ) ;
#10726=ORIENTED_EDGE ( 'NONE', *, *, #20965, .T. ) ;
#10738=ORIENTED_EDGE ( 'NONE', *, *, #20717, .T. ) ;
#10744=EDGE_CURVE ( 'NONE', #13013, #7142, #21112, .T. ) ;
#10765=ORIENTED_EDGE ( 'NONE', *, *, #16040, .T. ) ;
#10773=DIRECTION ( 'NONE',  ( -0.000000000000000000, 1.000000000000000000, 0.000000000000000000 ) ) ;
#10775=VERTEX_POINT ( 'NONE', #8785 ) ;
#10782=ADVANCED_FACE ( 'NONE', ( #10353 ), #17435, .T. ) ;
#10787=AXIS2_PLACEMENT_3D ( 'NONE', #6060, #6274, #2861 ) ;
#10788=ORIENTED_EDGE ( 'NONE', *, *, #3563, .T. ) ;
#10793=CARTESIAN_POINT ( 'NONE',  ( 21.43124999999999858, 16.27314499999999953, 8.731249999999999289 ) ) ;
#10798=VERTEX_POINT ( 'NONE', #8575 ) ;
#10803=VECTOR ( 'NONE', #11969, 1000.000000000000000 ) ;
#10806=ADVANCED_FACE ( 'NONE', ( #17096 ), #18959, .T. ) ;
#10807=CARTESIAN_POINT ( 'NONE',  ( 55.56250000000000000, 32.54502000000000095, -10.31874999999999964 ) ) ;
#10811=CARTESIAN_POINT ( 'NONE',  ( 65.90927232300019512, 1.984375000000000000, -13.30734117861468135 ) ) ;
#10815=CARTESIAN_POINT ( 'NONE',  ( 21.03437500000000071, 32.54502000000000095, 5.159374999999999822 ) ) ;
#10818=ORIENTED_EDGE ( 'NONE', *, *, #16672, .T. ) ;
#10820=ORIENTED_EDGE ( 'NONE', *, *, #14699, .T. ) ;
#10822=CARTESIAN_POINT ( 'NONE',  ( -1.724236557342190057, 0.000000000000000000, 8.786659759980359752 ) ) ;
#10823=DIRECTION ( 'NONE',  ( 0.000000000000000000, 1.000000000000000000, 0.000000000000000000 ) ) ;
#10830=DIRECTION ( 'NONE',  ( 0.000000000000000000, -1.000000000000000000, 0.000000000000000000 ) ) ;
#10831=CARTESIAN_POINT ( 'NONE',  ( 0.02083138522551555155, 20.24316500000000119, 7.210477125664100484 ) ) ;
#10840=ORIENTED_EDGE ( 'NONE', *, *, #311, .F. ) ;
#10844=CARTESIAN_POINT ( 'NONE',  ( 30.33489826846160398, 0.000000000000000000, -2.417033907079745525 ) ) ;
#10852=CARTESIAN_POINT ( 'NONE',  ( 24.60624999999999929, 16.27314499999999953, 8.731249999999999289 ) ) ;
#10856=PLANE ( 'NONE',  #2585 ) ;
#10859=DIRECTION ( 'NONE',  ( 0.000000000000000000, -1.000000000000000000, 0.000000000000000000 ) ) ;
#10863=CARTESIAN_POINT ( 'NONE',  ( 26.59062499828754866, 30.56080374999745075, 10.71562494918373964 ) ) ;
#10870=ORIENTED_EDGE ( 'NONE', *, *, #896, .T. ) ;
#10890=LINE ( 'NONE', #2604, #15901 ) ;
#10895=DIRECTION ( 'NONE',  ( 1.000000000000000000, 0.000000000000000000, 0.000000000000000000 ) ) ;
#10897=VECTOR ( 'NONE', #11986, 1000.000000000000000 ) ;
#10902=EDGE_CURVE ( 'NONE', #2714, #2722, #12622, .T. ) ;
#10906=CARTESIAN_POINT ( 'NONE',  ( 29.76562500000000000, 0.000000000000000000, -4.317999999999999616 ) ) ;
#10909=CYLINDRICAL_SURFACE ( 'NONE', #18448, 9.524999999999998579 ) ;
#10912=EDGE_LOOP ( 'NONE', ( #2948, #13948, #8419, #8169 ) ) ;
#10916=VERTEX_POINT ( 'NONE', #6138 ) ;
#10930=DIRECTION ( 'NONE',  ( 0.000000000000000000, 1.000000000000000000, 0.000000000000000000 ) ) ;
#10934=CARTESIAN_POINT ( 'NONE',  ( 6.585898268469219552, 32.54502000000000095, 4.694966092919240275 ) ) ;
#10935=DIRECTION ( 'NONE',  ( 1.000000000000000000, 0.000000000000000000, 0.000000000000000000 ) ) ;
#10937=ORIENTED_EDGE ( 'NONE', *, *, #21306, .F. ) ;
#10943=ORIENTED_EDGE ( 'NONE', *, *, #21018, .F. ) ;
#10953=EDGE_CURVE ( 'NONE', #395, #12583, #16012, .T. ) ;
#10966=FACE_BOUND ( 'NONE', #3829, .T. ) ;
#10969=ORIENTED_EDGE ( 'NONE', *, *, #17925, .F. ) ;
#10970=DIRECTION ( 'NONE',  ( -0.2868778675745010664, 0.000000000000000000, -0.9579671649362032637 ) ) ;
#10974=CARTESIAN_POINT ( 'NONE',  ( 28.78027906680959802, 1.604082891229885011, 10.67911709002892096 ) ) ;
#10978=AXIS2_PLACEMENT_3D ( 'NONE', #13572, #5147, #10231 ) ;
#10988=AXIS2_PLACEMENT_3D ( 'NONE', #8111, #16438, #4384 ) ;
#10998=ORIENTED_EDGE ( 'NONE', *, *, #9921, .F. ) ;
#11000=DIRECTION ( 'NONE',  ( 0.8334497143791951279, 0.000000000000000000, 0.5525953072558960066 ) ) ;
#11004=ORIENTED_EDGE ( 'NONE', *, *, #15072, .T. ) ;
#11005=FACE_BOUND ( 'NONE', #10656, .T. ) ;
#11012=CARTESIAN_POINT ( 'NONE',  ( 49.16323787629939801, -42.42568807200000691, -27.09503225884920141 ) ) ;
#11015=VERTEX_POINT ( 'NONE', #9772 ) ;
#11021=VECTOR ( 'NONE', #4751, 1000.000000000000000 ) ;
#11023=CARTESIAN_POINT ( 'NONE',  ( -12.30312499999999964, 2.380615000000000148, 8.335010000000000474 ) ) ;
#11027=ORIENTED_EDGE ( 'NONE', *, *, #21423, .F. ) ;
#11043=CARTESIAN_POINT ( 'NONE',  ( 71.04062499999999147, 0.000000000000000000, -10.31874999999999964 ) ) ;
#11048=ORIENTED_EDGE ( 'NONE', *, *, #7340, .T. ) ;
#11051=FACE_OUTER_BOUND ( 'NONE', #11484, .T. ) ;
#11053=VECTOR ( 'NONE', #14821, 1000.000000000000000 ) ;
#11058=DIRECTION ( 'NONE',  ( 0.000000000000000000, 1.000000000000000000, 0.000000000000000000 ) ) ;
#11062=ORIENTED_EDGE ( 'NONE', *, *, #11801, .T. ) ;
#11065=CIRCLE ( 'NONE', #6099, 3.968750000000000000 ) ;
#11075=CARTESIAN_POINT ( 'NONE',  ( -23.01875000000000071, 32.54502000000000095, -10.31874999999999964 ) ) ;
#11081=CARTESIAN_POINT ( 'NONE',  ( 1.268730000000000135, 23.41816500000000190, 10.65596716962832069 ) ) ;
#11088=ORIENTED_EDGE ( 'NONE', *, *, #11108, .F. ) ;
#11093=DIRECTION ( 'NONE',  ( 0.000000000000000000, -1.000000000000000000, 0.000000000000000000 ) ) ;
#11096=DIRECTION ( 'NONE',  ( 1.000000000000000000, 0.000000000000000000, 0.000000000000000000 ) ) ;
#11097=AXIS2_PLACEMENT_3D ( 'NONE', #19674, #21441, #6299 ) ;
#11101=CARTESIAN_POINT ( 'NONE',  ( 65.51436440461340283, 30.56064500000000095, -12.87863775929475985 ) ) ;
#11105=ADVANCED_FACE ( 'NONE', ( #8759 ), #18608, .T. ) ;
#11108=EDGE_CURVE ( 'NONE', #5953, #19328, #259, .T. ) ;
#11130=PLANE ( 'NONE',  #12273 ) ;
#11142=VERTEX_POINT ( 'NONE', #8432 ) ;
#11160=VERTEX_POINT ( 'NONE', #10440 ) ;
#11163=DIRECTION ( 'NONE',  ( -1.000000000000000000, 0.000000000000000000, 0.000000000000000000 ) ) ;
#11166=EDGE_LOOP ( 'NONE', ( #18415, #5936, #8428, #8249, #2638, #9321 ) ) ;
#11173=EDGE_CURVE ( 'NONE', #21060, #16032, #11607, .T. ) ;
#11180=AXIS2_PLACEMENT_3D ( 'NONE', #18493, #3254, #10428 ) ;
#11184=FACE_OUTER_BOUND ( 'NONE', #17643, .T. ) ;
#11190=CARTESIAN_POINT ( 'NONE',  ( 29.12736005702520359, 1.738817766846714852, 10.70064947183834114 ) ) ;
#11195=ORIENTED_EDGE ( 'NONE', *, *, #19050, .F. ) ;
#11212=ORIENTED_EDGE ( 'NONE', *, *, #14399, .T. ) ;
#11215=EDGE_LOOP ( 'NONE', ( #14781, #8603, #23, #21764 ) ) ;
#11219=DIRECTION ( 'NONE',  ( 0.1831666983862991482, 0.000000000000000000, -0.9830818687180954418 ) ) ;
#11220=ORIENTED_EDGE ( 'NONE', *, *, #17206, .F. ) ;
#11234=ORIENTED_EDGE ( 'NONE', *, *, #7193, .F. ) ;
#11236=CARTESIAN_POINT ( 'NONE',  ( -1.345424459097947834, 12.30439499999999953, 2.648158502653860324 ) ) ;
#11238=ORIENTED_EDGE ( 'NONE', *, *, #6431, .T. ) ;
#11245=EDGE_CURVE ( 'NONE', #7389, #12461, #6747, .T. ) ;
#11246=ORIENTED_EDGE ( 'NONE', *, *, #14399, .F. ) ;
#11258=ORIENTED_EDGE ( 'NONE', *, *, #21280, .F. ) ;
#11261=CARTESIAN_POINT ( 'NONE',  ( -12.30312499999999964, 1.984057500000000251, 10.71562499999999929 ) ) ;
#11263=VECTOR ( 'NONE', #12098, 1000.000000000000000 ) ;
#11285=DIRECTION ( 'NONE',  ( -0.3449240378348910063, 0.000000000000000000, 0.9386306025927743102 ) ) ;
#11288=CARTESIAN_POINT ( 'NONE',  ( 0.02083138522551555155, 20.24316500000000119, 7.210477125664100484 ) ) ;
#11289=CARTESIAN_POINT ( 'NONE',  ( 21.03437500000000071, 32.54502000000000095, 5.159374999999999822 ) ) ;
#11292=CARTESIAN_POINT ( 'NONE',  ( -29.36874999999999858, 30.56064500000000095, -3.968750000000000000 ) ) ;
#11299=CARTESIAN_POINT ( 'NONE',  ( 28.13664483251599790, 1.437813487382768152, 10.63918692494910090 ) ) ;
#11302=EDGE_CURVE ( 'NONE', #5275, #2212, #12677, .T. ) ;
#11306=DIRECTION ( 'NONE',  ( 0.8606571039906124598, -0.5091849853938075210, 0.000000000000000000 ) ) ;
#11310=AXIS2_PLACEMENT_3D ( 'NONE', #9568, #13026, #14795 ) ;
#11320=VECTOR ( 'NONE', #19396, 1000.000000000000000 ) ;
#11330=CIRCLE ( 'NONE', #7744, 2.381250000000001421 ) ;
#11339=CIRCLE ( 'NONE', #14896, 25.00312500000000426 ) ;
#11341=ORIENTED_EDGE ( 'NONE', *, *, #7933, .F. ) ;
#11344=CARTESIAN_POINT ( 'NONE',  ( 1.952969610814715207, 9.129395000000000593, 6.747510000000000119 ) ) ;
#11350=DIRECTION ( 'NONE',  ( 0.8624408385128676802, 0.5061578805720818863, 0.000000000000000000 ) ) ;
#11358=DIRECTION ( 'NONE',  ( -0.2868778675745011220, 0.000000000000000000, -0.9579671649362033747 ) ) ;
#11359=EDGE_LOOP ( 'NONE', ( #16656, #19966, #3418, #5445 ) ) ;
#11361=EDGE_LOOP ( 'NONE', ( #12515, #15563, #17433, #16246 ) ) ;
#11363=EDGE_LOOP ( 'NONE', ( #658, #3751, #6857, #8610 ) ) ;
#11382=CARTESIAN_POINT ( 'NONE',  ( 66.03921914090641110, 30.56064500000000095, -11.33033647675950029 ) ) ;
#11384=ORIENTED_EDGE ( 'NONE', *, *, #10240, .T. ) ;
#11392=CYLINDRICAL_SURFACE ( 'NONE', #12388, 0.3962400000000008138 ) ;
#11399=CARTESIAN_POINT ( 'NONE',  ( 67.79270099634359781, 30.56064500000000095, -13.76558698117381851 ) ) ;
#11400=DIRECTION ( 'NONE',  ( 1.000000000000000000, 0.000000000000000000, 0.000000000000000000 ) ) ;
#11403=CARTESIAN_POINT ( 'NONE',  ( 1.952969610814715207, 23.41816500000000190, 6.747510000000000119 ) ) ;
#11406=CARTESIAN_POINT ( 'NONE',  ( 46.03750000000000142, 0.000000000000000000, -10.31874999999999964 ) ) ;
#11419=DIRECTION ( 'NONE',  ( -0.06191955310929833645, 0.000000000000000000, 0.9980811434661738257 ) ) ;
#11421=DIRECTION ( 'NONE',  ( 0.000000000000000000, 0.000000000000000000, 1.000000000000000000 ) ) ;
#11422=AXIS2_PLACEMENT_3D ( 'NONE', #12630, #2113, #17496 ) ;
#11427=ADVANCED_FACE ( 'NONE', ( #1094 ), #19559, .F. ) ;
#11438=CARTESIAN_POINT ( 'NONE',  ( -17.46249999999999858, 16.27314499999999953, 10.71562499999999929 ) ) ;
#11444=CARTESIAN_POINT ( 'NONE',  ( 29.19635173153840313, 0.000000000000000000, -6.218966092919240296 ) ) ;
#11450=CARTESIAN_POINT ( 'NONE',  ( 46.03750000000000142, 30.56064500000000095, -10.31874999999999964 ) ) ;
#11451=VERTEX_POINT ( 'NONE', #17580 ) ;
#11454=PRODUCT_DEFINITION_SHAPE ( 'NONE', 'NONE',  #1012 ) ;
#11462=CARTESIAN_POINT ( 'NONE',  ( 2.063750000000000195, 30.56064500000000095, -19.71675000000000111 ) ) ;
#11472=ORIENTED_EDGE ( 'NONE', *, *, #14413, .T. ) ;
#11474=EDGE_LOOP ( 'NONE', ( #15324, #14012 ) ) ;
#11477=ORIENTED_EDGE ( 'NONE', *, *, #10902, .F. ) ;
#11479=EDGE_CURVE ( 'NONE', #2212, #5275, #2076, .T. ) ;
#11482=DIRECTION ( 'NONE',  ( 0.000000000000000000, -1.000000000000000000, 0.000000000000000000 ) ) ;
#11484=EDGE_LOOP ( 'NONE', ( #12482, #6339, #7608, #4316 ) ) ;
#11487=CARTESIAN_POINT ( 'NONE',  ( -29.36874999999999858, 2.380615000000000148, 8.731249999999999289 ) ) ;
#11489=VERTEX_POINT ( 'NONE', #17809 ) ;
#11494=AXIS2_PLACEMENT_3D ( 'NONE', #20507, #21152, #9541 ) ;
#11495=ORIENTED_EDGE ( 'NONE', *, *, #16678, .F. ) ;
#11496=CARTESIAN_POINT ( 'NONE',  ( -17.46249999999999858, 0.000000000000000000, 0.000000000000000000 ) ) ;
#11511=FACE_OUTER_BOUND ( 'NONE', #2892, .T. ) ;
#11513=ORIENTED_EDGE ( 'NONE', *, *, #4721, .F. ) ;
#11522=EDGE_CURVE ( 'NONE', #1449, #7354, #14825, .T. ) ;
#11526=EDGE_CURVE ( 'NONE', #18861, #7013, #7018, .T. ) ;
#11530=FACE_OUTER_BOUND ( 'NONE', #21077, .T. ) ;
#11548=ORIENTED_EDGE ( 'NONE', *, *, #7340, .F. ) ;
#11564=VERTEX_POINT ( 'NONE', #2869 ) ;
#11570=CARTESIAN_POINT ( 'NONE',  ( 54.11611804786240043, 1.984375000000000000, -30.58983753981140197 ) ) ;
#11577=ADVANCED_FACE ( 'NONE', ( #11595 ), #21536, .T. ) ;
#11580=ORIENTED_EDGE ( 'NONE', *, *, #21663, .F. ) ;
#11581=DIRECTION ( 'NONE',  ( 0.000000000000000000, -1.000000000000000000, 0.000000000000000000 ) ) ;
#11594=LINE ( 'NONE', #18008, #10305 ) ;
#11595=FACE_OUTER_BOUND ( 'NONE', #18957, .T. ) ;
#11600=VERTEX_POINT ( 'NONE', #9711 ) ;
#11603=FACE_OUTER_BOUND ( 'NONE', #20173, .T. ) ;
#11607=CIRCLE ( 'NONE', #1349, 0.3962400000000008138 ) ;
#11610=DIRECTION ( 'NONE',  ( 0.000000000000000000, 1.000000000000000000, 0.000000000000000000 ) ) ;
#11616=DIRECTION ( 'NONE',  ( 0.000000000000000000, -1.000000000000000000, 0.000000000000000000 ) ) ;
#11622=DIRECTION ( 'NONE',  ( 1.000000000000000000, 0.000000000000000000, 0.000000000000000000 ) ) ;
#11624=VERTEX_POINT ( 'NONE', #10477 ) ;
#11631=CARTESIAN_POINT ( 'NONE',  ( 29.19635173153840313, 1.984375000000000000, -6.218966092919240296 ) ) ;
#11644=ORIENTED_EDGE ( 'NONE', *, *, #16040, .F. ) ;
#11654=DIRECTION ( 'NONE',  ( 0.000000000000000000, -1.000000000000000000, 0.000000000000000000 ) ) ;
#11655=ORIENTED_EDGE ( 'NONE', *, *, #19326, .T. ) ;
#11671=VECTOR ( 'NONE', #21185, 1000.000000000000000 ) ;
#11674=CARTESIAN_POINT ( 'NONE',  ( -2.607150795738780058, 32.54502000000000095, 8.731885000000000119 ) ) ;
#11675=ORIENTED_EDGE ( 'NONE', *, *, #5793, .T. ) ;
#11678=EDGE_CURVE ( 'NONE', #1714, #11160, #8778, .T. ) ;
#11680=PLANE ( 'NONE',  #16983 ) ;
#11693=LINE ( 'NONE', #15468, #19845 ) ;
#11694=ADVANCED_FACE ( 'NONE', ( #20400 ), #11917, .F. ) ;
#11696=DIRECTION ( 'NONE',  ( 0.000000000000000000, 0.000000000000000000, 1.000000000000000000 ) ) ;
#11700=AXIS2_PLACEMENT_3D ( 'NONE', #16900, #1748, #15899 ) ;
#11701=ORIENTED_EDGE ( 'NONE', *, *, #7265, .F. ) ;
#11712=ORIENTED_EDGE ( 'NONE', *, *, #21811, .T. ) ;
#11715=LINE ( 'NONE', #19887, #1433 ) ;
#11716=ORIENTED_EDGE ( 'NONE', *, *, #7092, .T. ) ;
#11719=AXIS2_PLACEMENT_3D ( 'NONE', #6539, #3217, #9629 ) ;
#11731=DIRECTION ( 'NONE',  ( 1.000000000000000000, 0.000000000000000000, 0.000000000000000000 ) ) ;
#11736=ORIENTED_EDGE ( 'NONE', *, *, #18905, .T. ) ;
#11739=CYLINDRICAL_SURFACE ( 'NONE', #7475, 2.381250000000001421 ) ;
#11741=ORIENTED_EDGE ( 'NONE', *, *, #10430, .T. ) ;
#11742=AXIS2_PLACEMENT_3D ( 'NONE', #17430, #17195, #12458 ) ;
#11745=FACE_OUTER_BOUND ( 'NONE', #11363, .T. ) ;
#11746=CARTESIAN_POINT ( 'NONE',  ( -3.929154139288399961, 23.41816500000000190, 0.9374890779182719625 ) ) ;
#11750=AXIS2_PLACEMENT_3D ( 'NONE', #291, #13369, #4846 ) ;
#11763=EDGE_LOOP ( 'NONE', ( #3959, #15342 ) ) ;
#11799=VECTOR ( 'NONE', #7965, 1000.000000000000000 ) ;
#11801=EDGE_CURVE ( 'NONE', #5219, #4077, #9131, .T. ) ;
#11808=EDGE_CURVE ( 'NONE', #966, #13820, #17269, .T. ) ;
#11816=DIRECTION ( 'NONE',  ( 0.9966381950048638361, 0.000000000000000000, -0.08192867786951699149 ) ) ;
#11817=DIRECTION ( 'NONE',  ( 1.000000000000000000, 0.000000000000000000, 0.000000000000000000 ) ) ;
#11818=LINE ( 'NONE', #5165, #18403 ) ;
#11821=ORIENTED_EDGE ( 'NONE', *, *, #1891, .F. ) ;
#11822=EDGE_LOOP ( 'NONE', ( #18936, #17794 ) ) ;
#11829=EDGE_LOOP ( 'NONE', ( #17002, #11246, #21403, #21210 ) ) ;
#11856=DIRECTION ( 'NONE',  ( -0.7776383362760928009, 0.000000000000000000, 0.6287118719681937806 ) ) ;
#11864=CARTESIAN_POINT ( 'NONE',  ( -160.2647810241784896, 30.56064500000000095, 10.71562489836746046 ) ) ;
#11872=VERTEX_POINT ( 'NONE', #3742 ) ;
#11879=DIRECTION ( 'NONE',  ( 0.000000000000000000, 0.000000000000000000, 1.000000000000000000 ) ) ;
#11909=CARTESIAN_POINT ( 'NONE',  ( -29.36874999999999858, 23.41816500000000190, 0.000000000000000000 ) ) ;
#11915=EDGE_CURVE ( 'NONE', #1449, #6627, #8079, .T. ) ;
#11916=DIRECTION ( 'NONE',  ( 0.000000000000000000, 0.000000000000000000, 1.000000000000000000 ) ) ;
#11917=CYLINDRICAL_SURFACE ( 'NONE', #12335, 3.175000000000000711 ) ;
#11922=VECTOR ( 'NONE', #10273, 1000.000000000000000 ) ;
#11924=ORIENTED_EDGE ( 'NONE', *, *, #8819, .T. ) ;
#11929=ADVANCED_FACE ( 'NONE', ( #2293 ), #4400, .T. ) ;
#11933=FACE_OUTER_BOUND ( 'NONE', #6864, .T. ) ;
#11940=DIRECTION ( 'NONE',  ( -0.2868778675745008999, 0.000000000000000000, -0.9579671649362034858 ) ) ;
#11956=DIRECTION ( 'NONE',  ( 0.000000000000000000, -1.000000000000000000, 0.000000000000000000 ) ) ;
#11959=DIRECTION ( 'NONE',  ( -0.6287118719681937806, 0.000000000000000000, -0.7776383362760928009 ) ) ;
#11961=CARTESIAN_POINT ( 'NONE',  ( 29.37436411451823304, 31.72299998434776569, 10.71597283099095499 ) ) ;
#11969=DIRECTION ( 'NONE',  ( 1.000000000000000000, 0.000000000000000000, 0.000000000000000000 ) ) ;
#11972=EDGE_CURVE ( 'NONE', #9795, #13402, #17663, .T. ) ;
#11980=CARTESIAN_POINT ( 'NONE',  ( 26.59062499999999929, 26.59189500000000095, 10.71562499999999929 ) ) ;
#11982=DIRECTION ( 'NONE',  ( 0.000000000000000000, 1.000000000000000000, 0.000000000000000000 ) ) ;
#11983=ORIENTED_EDGE ( 'NONE', *, *, #16573, .F. ) ;
#11986=DIRECTION ( 'NONE',  ( 0.000000000000000000, 0.000000000000000000, 1.000000000000000000 ) ) ;
#11987=AXIS2_PLACEMENT_3D ( 'NONE', #528, #7277, #14038 ) ;
#11989=VECTOR ( 'NONE', #14238, 1000.000000000000000 ) ;
#11993=AXIS2_PLACEMENT_3D ( 'NONE', #15877, #7450, #20941 ) ;
#11999=VERTEX_POINT ( 'NONE', #12453 ) ;
#12010=AXIS2_PLACEMENT_3D ( 'NONE', #16208, #17421, #5804 ) ;
#12025=DIRECTION ( 'NONE',  ( 0.000000000000000000, 1.000000000000000000, 0.000000000000000000 ) ) ;
#12030=EDGE_LOOP ( 'NONE', ( #7234, #18086, #9237, #18218 ) ) ;
#12037=VERTEX_POINT ( 'NONE', #14440 ) ;
#12048=DIRECTION ( 'NONE',  ( 0.8334497143791951279, 0.000000000000000000, 0.5525953072558960066 ) ) ;
#12054=ORIENTED_EDGE ( 'NONE', *, *, #6904, .T. ) ;
#12057=LINE ( 'NONE', #17026, #19128 ) ;
#12065=VERTEX_POINT ( 'NONE', #2380 ) ;
#12086=CARTESIAN_POINT ( 'NONE',  ( -3.929154139288399961, 9.129395000000000593, 0.9374890779182719625 ) ) ;
#12088=DIRECTION ( 'NONE',  ( 0.000000000000000000, 1.000000000000000000, 0.000000000000000000 ) ) ;
#12098=DIRECTION ( 'NONE',  ( 0.000000000000000000, 1.000000000000000000, 0.000000000000000000 ) ) ;
#12108=ORIENTED_EDGE ( 'NONE', *, *, #1311, .T. ) ;
#12113=CARTESIAN_POINT ( 'NONE',  ( 21.03437500000000071, 32.54502000000000095, 5.159374999999999822 ) ) ;
#12118=ORIENTED_EDGE ( 'NONE', *, *, #5034, .F. ) ;
#12123=CARTESIAN_POINT ( 'NONE',  ( 66.87634738983680904, 0.000000000000000000, 3.497859541731999755 ) ) ;
#12142=CARTESIAN_POINT ( 'NONE',  ( -12.30312499999999964, 2.380615000000000148, 8.731249999999999289 ) ) ;
#12147=DIRECTION ( 'NONE',  ( -1.000000000000000000, 0.000000000000000000, 0.000000000000000000 ) ) ;
#12150=VECTOR ( 'NONE', #17135, 1000.000000000000000 ) ;
#12159=CIRCLE ( 'NONE', #11097, 0.3962400000000008138 ) ;
#12179=VERTEX_POINT ( 'NONE', #13112 ) ;
#12180=AXIS2_PLACEMENT_3D ( 'NONE', #323, #8497, #15279 ) ;
#12181=ORIENTED_EDGE ( 'NONE', *, *, #4496, .F. ) ;
#12188=EDGE_CURVE ( 'NONE', #9189, #10775, #6236, .T. ) ;
#12198=DIRECTION ( 'NONE',  ( 0.000000000000000000, 1.000000000000000000, 0.000000000000000000 ) ) ;
#12199=CYLINDRICAL_SURFACE ( 'NONE', #7964, 0.3962399999999999811 ) ;
#12207=ORIENTED_EDGE ( 'NONE', *, *, #691, .F. ) ;
#12209=AXIS2_PLACEMENT_3D ( 'NONE', #3903, #15193, #15310 ) ;
#12216=ORIENTED_EDGE ( 'NONE', *, *, #21352, .F. ) ;
#12224=ORIENTED_EDGE ( 'NONE', *, *, #2790, .F. ) ;
#12234=ORIENTED_EDGE ( 'NONE', *, *, #5876, .F. ) ;
#12245=CARTESIAN_POINT ( 'NONE',  ( 46.03750000000000142, 0.000000000000000000, -10.31874999999999964 ) ) ;
#12250=LINE ( 'NONE', #12479, #7729 ) ;
#12251=DIRECTION ( 'NONE',  ( 1.000000000000000000, 0.000000000000000000, 0.000000000000000000 ) ) ;
#12255=EDGE_LOOP ( 'NONE', ( #5805, #20486, #16004, #3663, #21510 ) ) ;
#12273=AXIS2_PLACEMENT_3D ( 'NONE', #6036, #16022, #7596 ) ;
#12276=CARTESIAN_POINT ( 'NONE',  ( -29.36874999999999858, 30.56128000000000000, 8.731885000000000119 ) ) ;
#12297=CARTESIAN_POINT ( 'NONE',  ( -29.36874999999999858, 1.984375000000000000, -3.968750000000000000 ) ) ;
#12301=CYLINDRICAL_SURFACE ( 'NONE', #12209, 0.3962399999999988154 ) ;
#12305=DIRECTION ( 'NONE',  ( 0.000000000000000000, 1.000000000000000000, 0.000000000000000000 ) ) ;
#12314=ADVANCED_FACE ( 'NONE', ( #21712 ), #6566, .F. ) ;
#12315=CARTESIAN_POINT ( 'NONE',  ( 2.063750000000000195, 1.984375000000000000, 8.335010000000000474 ) ) ;
#12324=AXIS2_PLACEMENT_3D ( 'NONE', #19595, #4461, #1132 ) ;
#12328=EDGE_CURVE ( 'NONE', #20613, #2429, #21810, .T. ) ;
#12335=AXIS2_PLACEMENT_3D ( 'NONE', #18873, #8922, #12251 ) ;
#12343=AXIS2_PLACEMENT_3D ( 'NONE', #14915, #16663, #16773 ) ;
#12356=ORIENTED_EDGE ( 'NONE', *, *, #18913, .T. ) ;
#12364=ORIENTED_EDGE ( 'NONE', *, *, #6140, .T. ) ;
#12365=EDGE_LOOP ( 'NONE', ( #17978, #10574, #5887, #986 ) ) ;
#12382=EDGE_CURVE ( 'NONE', #19328, #395, #16943, .T. ) ;
#12388=AXIS2_PLACEMENT_3D ( 'NONE', #13490, #21874, #18137 ) ;
#12408=CIRCLE ( 'NONE', #7798, 1.983739999999999393 ) ;
#12417=DIRECTION ( 'NONE',  ( 0.9876802608827758290, 0.000000000000000000, -0.1564854698127972066 ) ) ;
#12420=DIRECTION ( 'NONE',  ( 0.000000000000000000, 1.000000000000000000, 0.000000000000000000 ) ) ;
#12424=DIRECTION ( 'NONE',  ( 1.000000000000000000, 0.000000000000000000, 0.000000000000000000 ) ) ;
#12433=ORIENTED_EDGE ( 'NONE', *, *, #4022, .T. ) ;
#12436=CARTESIAN_POINT ( 'NONE',  ( 71.04062499999999147, 1.984375000000000000, -10.31874999999999964 ) ) ;
#12451=ORIENTED_EDGE ( 'NONE', *, *, #2047, .T. ) ;
#12453=CARTESIAN_POINT ( 'NONE',  ( 54.11611804786240043, 30.56064500000000095, -30.58983753981140197 ) ) ;
#12458=DIRECTION ( 'NONE',  ( 1.000000000000000000, 0.000000000000000000, 0.000000000000000000 ) ) ;
#12460=CARTESIAN_POINT ( 'NONE',  ( 29.19635173153840313, 32.54502000000000095, -6.218966092919240296 ) ) ;
#12461=VERTEX_POINT ( 'NONE', #9279 ) ;
#12472=AXIS2_PLACEMENT_3D ( 'NONE', #16789, #1736, #8159 ) ;
#12474=LINE ( 'NONE', #2051, #793 ) ;
#12477=ORIENTED_EDGE ( 'NONE', *, *, #9543, .T. ) ;
#12479=CARTESIAN_POINT ( 'NONE',  ( 49.41235866845560309, 30.56064500000000095, -26.78690084448080100 ) ) ;
#12481=DIRECTION ( 'NONE',  ( -0.9579671649362032637, 0.000000000000000000, 0.2868778675745010664 ) ) ;
#12482=ORIENTED_EDGE ( 'NONE', *, *, #14796, .F. ) ;
#12494=EDGE_CURVE ( 'NONE', #5923, #10689, #9162, .T. ) ;
#12495=LINE ( 'NONE', #19219, #14580 ) ;
#12498=CARTESIAN_POINT ( 'NONE',  ( 1.268730000000000135, 23.41816500000000190, 8.609509071587499562 ) ) ;
#12508=DIRECTION ( 'NONE',  ( 1.000000000000000000, 0.000000000000000000, 0.000000000000000000 ) ) ;
#12513=AXIS2_PLACEMENT_3D ( 'NONE', #15904, #12575, #5477 ) ;
#12515=ORIENTED_EDGE ( 'NONE', *, *, #316, .F. ) ;
#12516=EDGE_CURVE ( 'NONE', #5609, #9456, #7735, .T. ) ;
#12521=DIRECTION ( 'NONE',  ( 0.000000000000000000, 1.000000000000000000, 0.000000000000000000 ) ) ;
#12536=AXIS2_PLACEMENT_3D ( 'NONE', #7454, #14112, #14228 ) ;
#12542=EDGE_CURVE ( 'NONE', #9016, #8141, #14740, .T. ) ;
#12552=AXIS2_PLACEMENT_3D ( 'NONE', #10162, #18462, #1977 ) ;
#12555=FACE_OUTER_BOUND ( 'NONE', #2708, .T. ) ;
#12557=DIRECTION ( 'NONE',  ( 0.000000000000000000, -1.000000000000000000, 0.000000000000000000 ) ) ;
#12561=ORIENTED_EDGE ( 'NONE', *, *, #14538, .T. ) ;
#12572=DIRECTION ( 'NONE',  ( -1.000000000000000000, 0.000000000000000000, 0.000000000000000000 ) ) ;
#12575=DIRECTION ( 'NONE',  ( 1.000000000000000000, 0.000000000000000000, 0.000000000000000000 ) ) ;
#12583=VERTEX_POINT ( 'NONE', #2546 ) ;
#12591=ORIENTED_EDGE ( 'NONE', *, *, #6160, .F. ) ;
#12596=VERTEX_POINT ( 'NONE', #17695 ) ;
#12598=CARTESIAN_POINT ( 'NONE',  ( 10.00557973814771984, 0.1597379260826150282, 9.514361097518639454 ) ) ;
#12608=ORIENTED_EDGE ( 'NONE', *, *, #6603, .F. ) ;
#12620=LINE ( 'NONE', #7636, #4858 ) ;
#12622=B_SPLINE_CURVE_WITH_KNOTS ( 'NONE', 3,
 ( #15789, #21283, #7362, #20961, #19519, #14348, #20835, #726 ),
 .UNSPECIFIED., .F., .F.,
 ( 4, 2, 2, 4 ),
 ( 0.000000000000000000, 0.2499999999999988898, 0.4999999999999977796, 1.000000000000000000 ),
 .UNSPECIFIED. ) ;
#12626=CARTESIAN_POINT ( 'NONE',  ( 29.36887348155339694, 30.56064500123875050, 10.71562877576799977 ) ) ;
#12627=AXIS2_PLACEMENT_3D ( 'NONE', #6522, #16797, #1534 ) ;
#12630=CARTESIAN_POINT ( 'NONE',  ( 65.90927232300019512, -42.42568807200000691, -12.91110117861467899 ) ) ;
#12637=PLANE ( 'NONE',  #14866 ) ;
#12645=CARTESIAN_POINT ( 'NONE',  ( 25.20528082976425210, 1.004445366757521940, 10.45732921704471963 ) ) ;
#12650=PLANE ( 'NONE',  #2127 ) ;
#12651=CARTESIAN_POINT ( 'NONE',  ( -29.36874999999999858, 30.56064500000000095, 8.731249999999999289 ) ) ;
#12669=DIRECTION ( 'NONE',  ( 0.000000000000000000, 1.000000000000000000, 0.000000000000000000 ) ) ;
#12670=CARTESIAN_POINT ( 'NONE',  ( 54.11611804786240043, 32.54502000000000095, -30.58983753981140197 ) ) ;
#12672=CARTESIAN_POINT ( 'NONE',  ( -29.36874999999999858, 32.54502000000000095, 8.731885000000000119 ) ) ;
#12677=CIRCLE ( 'NONE', #8762, 3.968750000000000000 ) ;
#12682=CARTESIAN_POINT ( 'NONE',  ( 50.99913033092320092, 0.000000000000000000, -7.029081061492260751 ) ) ;
#12688=VERTEX_POINT ( 'NONE', #1424 ) ;
#12691=ORIENTED_EDGE ( 'NONE', *, *, #16959, .F. ) ;
#12701=ORIENTED_EDGE ( 'NONE', *, *, #8955, .T. ) ;
#12720=APPLICATION_CONTEXT ( 'automotive_design' ) ;
#12722=LINE ( 'NONE', #21326, #14566 ) ;
#12736=ADVANCED_FACE ( 'NONE', ( #5074 ), #8166, .F. ) ;
#12749=LINE ( 'NONE', #4227, #16993 ) ;
#12751=AXIS2_PLACEMENT_3D ( 'NONE', #8218, #14875, #17961 ) ;
#12755=ORIENTED_EDGE ( 'NONE', *, *, #14813, .T. ) ;
#12757=CARTESIAN_POINT ( 'NONE',  ( 21.23834649789565177, 0.6614900943270459743, 10.21122617957944101 ) ) ;
#12761=DIRECTION ( 'NONE',  ( 0.000000000000000000, 0.000000000000000000, 1.000000000000000000 ) ) ;
#12764=EDGE_CURVE ( 'NONE', #13849, #7932, #21542, .T. ) ;
#12765=FACE_OUTER_BOUND ( 'NONE', #5302, .T. ) ;
#12772=AXIS2_PLACEMENT_3D ( 'NONE', #4240, #21139, #2584 ) ;
#12779=DIRECTION ( 'NONE',  ( 0.000000000000000000, 0.000000000000000000, -1.000000000000000000 ) ) ;
#12785=ORIENTED_EDGE ( 'NONE', *, *, #665, .F. ) ;
#12798=EDGE_LOOP ( 'NONE', ( #7280, #7784 ) ) ;
#12805=CIRCLE ( 'NONE', #10302, 16.66874999999998508 ) ;
#12822=VERTEX_POINT ( 'NONE', #10844 ) ;
#12825=VERTEX_POINT ( 'NONE', #17592 ) ;
#12831=CARTESIAN_POINT ( 'NONE',  ( 65.64431122251959039, 1.984375000000000000, -11.29787305743958115 ) ) ;
#12836=DIRECTION ( 'NONE',  ( 0.000000000000000000, 1.000000000000000000, 0.000000000000000000 ) ) ;
#12841=ORIENTED_EDGE ( 'NONE', *, *, #2922, .F. ) ;
#12846=ORIENTED_EDGE ( 'NONE', *, *, #15634, .F. ) ;
#12848=EDGE_CURVE ( 'NONE', #11872, #18115, #12620, .T. ) ;
#12879=CARTESIAN_POINT ( 'NONE',  ( 65.47912282493159353, 0.000000000000000000, -13.30734117861468135 ) ) ;
#12885=CARTESIAN_POINT ( 'NONE',  ( 71.03963378001139972, 30.56064500000000095, -10.54138470677948014 ) ) ;
#12886=CARTESIAN_POINT ( 'NONE',  ( -13.49374999999999858, 0.000000000000000000, 0.000000000000000000 ) ) ;
#12892=VERTEX_POINT ( 'NONE', #295 ) ;
#12901=EDGE_CURVE ( 'NONE', #3881, #13013, #17202, .T. ) ;
#12910=EDGE_LOOP ( 'NONE', ( #4282, #12924, #7052, #5268 ) ) ;
#12917=EDGE_CURVE ( 'NONE', #2958, #8281, #8796, .T. ) ;
#12924=ORIENTED_EDGE ( 'NONE', *, *, #17206, .T. ) ;
#12926=EDGE_CURVE ( 'NONE', #11999, #9809, #6957, .T. ) ;
#12931=ORIENTED_EDGE ( 'NONE', *, *, #6729, .T. ) ;
#12939=LINE ( 'NONE', #14604, #17076 ) ;
#12948=DIRECTION ( 'NONE',  ( 0.000000000000000000, 0.000000000000000000, -1.000000000000000000 ) ) ;
#12950=DIRECTION ( 'NONE',  ( 0.000000000000000000, 1.000000000000000000, 0.000000000000000000 ) ) ;
#12963=LINE ( 'NONE', #2774, #11799 ) ;
#12967=EDGE_CURVE ( 'NONE', #10050, #7705, #9712, .T. ) ;
#12980=CARTESIAN_POINT ( 'NONE',  ( 31.75000000000000000, 0.000000000000000000, -4.317999999999999616 ) ) ;
#12985=LINE ( 'NONE', #16301, #16946 ) ;
#12991=CARTESIAN_POINT ( 'NONE',  ( 46.03750000000000142, 0.000000000000000000, -10.31874999999999964 ) ) ;
#12998=CARTESIAN_POINT ( 'NONE',  ( 2.063750000000000195, 2.380615000000000148, 8.335010000000000474 ) ) ;
#13009=CARTESIAN_POINT ( 'NONE',  ( 28.97711086133420366, 0.000000000000000000, -10.31874999999999964 ) ) ;
#13013=VERTEX_POINT ( 'NONE', #5259 ) ;
#13014=DIRECTION ( 'NONE',  ( 0.6287118719681975554, 0.000000000000000000, 0.7776383362760898033 ) ) ;
#13015=ORIENTED_EDGE ( 'NONE', *, *, #10215, .F. ) ;
#13026=DIRECTION ( 'NONE',  ( 0.000000000000000000, 1.000000000000000000, 0.000000000000000000 ) ) ;
#13029=CARTESIAN_POINT ( 'NONE',  ( -1.848761088705630051, 9.129395000000000593, 7.884515871828260636 ) ) ;
#13035=ORIENTED_EDGE ( 'NONE', *, *, #9921, .T. ) ;
#13038=VERTEX_POINT ( 'NONE', #6829 ) ;
#13040=EDGE_CURVE ( 'NONE', #17367, #13795, #20846, .T. ) ;
#13042=AXIS2_PLACEMENT_3D ( 'NONE', #11382, #16690, #8372 ) ;
#13046=DIRECTION ( 'NONE',  ( 0.000000000000000000, 0.000000000000000000, 1.000000000000000000 ) ) ;
#13048=FACE_OUTER_BOUND ( 'NONE', #4630, .T. ) ;
#13053=CARTESIAN_POINT ( 'NONE',  ( 29.36874999999999858, 0.000000000000000000, -10.31874999999999964 ) ) ;
#13055=VECTOR ( 'NONE', #2247, 1000.000000000000227 ) ;
#13064=DIRECTION ( 'NONE',  ( 1.000000000000000000, 0.000000000000000000, 0.000000000000000000 ) ) ;
#13072=VECTOR ( 'NONE', #18167, 1000.000000000000000 ) ;
#13080=CARTESIAN_POINT ( 'NONE',  ( 1.537498671273937578, 23.46184445063047974, 10.69425292771247449 ) ) ;
#13089=VERTEX_POINT ( 'NONE', #10807 ) ;
#13094=CARTESIAN_POINT ( 'NONE',  ( 1.268730000000000135, 24.21318500000000284, 8.731249999999999289 ) ) ;
#13111=AXIS2_PLACEMENT_3D ( 'NONE', #5047, #1186, #4731 ) ;
#13112=CARTESIAN_POINT ( 'NONE',  ( 67.40134256979101224, 0.000000000000000000, -13.30734117861468135 ) ) ;
#13113=EDGE_LOOP ( 'NONE', ( #15293, #6166, #8683, #17692 ) ) ;
#13120=FACE_OUTER_BOUND ( 'NONE', #4429, .T. ) ;
#13121=ADVANCED_FACE ( 'NONE', ( #4168 ), #11130, .T. ) ;
#13126=VECTOR ( 'NONE', #3154, 1000.000000000000227 ) ;
#13136=DIRECTION ( 'NONE',  ( -1.000000000000000000, 0.000000000000000000, 0.000000000000000000 ) ) ;
#13140=CIRCLE ( 'NONE', #14565, 2.381250000000001421 ) ;
#13153=EDGE_LOOP ( 'NONE', ( #1171, #5815, #2032, #20407 ) ) ;
#13162=ORIENTED_EDGE ( 'NONE', *, *, #1413, .F. ) ;
#13165=PLANE ( 'NONE',  #15640 ) ;
#13176=CARTESIAN_POINT ( 'NONE',  ( 65.64431122251959039, 0.000000000000000000, -11.29787305743958115 ) ) ;
#13187=LINE ( 'NONE', #8071, #19327 ) ;
#13191=DIRECTION ( 'NONE',  ( 0.000000000000000000, 1.000000000000000000, 0.000000000000000000 ) ) ;
#13205=CYLINDRICAL_SURFACE ( 'NONE', #20117, 1.983739999999999393 ) ;
#13210=DIRECTION ( 'NONE',  ( 0.000000000000000000, 0.000000000000000000, -1.000000000000000000 ) ) ;
#13221=ADVANCED_FACE ( 'NONE', ( #9886 ), #19847, .F. ) ;
#13222=ORIENTED_EDGE ( 'NONE', *, *, #11915, .T. ) ;
#13232=AXIS2_PLACEMENT_3D ( 'NONE', #11012, #4274, #7366 ) ;
#13253=ORIENTED_EDGE ( 'NONE', *, *, #11522, .F. ) ;
#13254=ORIENTED_EDGE ( 'NONE', *, *, #3589, .T. ) ;
#13266=VECTOR ( 'NONE', #6175, 1000.000000000000000 ) ;
#13272=ADVANCED_FACE ( 'NONE', ( #1498 ), #4722, .F. ) ;
#13274=DIRECTION ( 'NONE',  ( 0.8334497143791944618, 0.000000000000000000, 0.5525953072558966728 ) ) ;
#13275=CARTESIAN_POINT ( 'NONE',  ( 70.64340948846358970, 1.984375000000000000, -10.93409647675949969 ) ) ;
#13276=LINE ( 'NONE', #4524, #17015 ) ;
#13278=ORIENTED_EDGE ( 'NONE', *, *, #9567, .T. ) ;
#13283=AXIS2_PLACEMENT_3D ( 'NONE', #13755, #12088, #15420 ) ;
#13285=DIRECTION ( 'NONE',  ( 0.000000000000000000, 1.000000000000000000, 0.000000000000000000 ) ) ;
#13292=DIRECTION ( 'NONE',  ( 0.000000000000000000, 1.000000000000000000, 0.000000000000000000 ) ) ;
#13297=ADVANCED_FACE ( 'NONE', ( #21836 ), #2835, .F. ) ;
#13302=CARTESIAN_POINT ( 'NONE',  ( -4.157227781567939928, 9.924415000000001541, 0.1758860224507720060 ) ) ;
#13305=CARTESIAN_POINT ( 'NONE',  ( 21.03437500000000071, 32.54502000000000095, 5.159374999999999822 ) ) ;
#13311=CARTESIAN_POINT ( 'NONE',  ( 5.447351731530780228, 1.984375000000000000, 0.8930339070797439494 ) ) ;
#13312=DIRECTION ( 'NONE',  ( -0.06191955310929833645, 0.000000000000000000, 0.9980811434661738257 ) ) ;
#13322=CARTESIAN_POINT ( 'NONE',  ( 28.97711086133420366, -42.42568807200000691, -10.71499000000000024 ) ) ;
#13331=AXIS2_PLACEMENT_3D ( 'NONE', #19564, #4529, #11163 ) ;
#13345=DIRECTION ( 'NONE',  ( 0.000000000000000000, 1.000000000000000000, 0.000000000000000000 ) ) ;
#13353=ORIENTED_EDGE ( 'NONE', *, *, #11526, .F. ) ;
#13361=AXIS2_PLACEMENT_3D ( 'NONE', #18998, #17361, #15722 ) ;
#13369=DIRECTION ( 'NONE',  ( 0.000000000000000000, -1.000000000000000000, 0.000000000000000000 ) ) ;
#13370=PLANE ( 'NONE',  #15746 ) ;
#13374=DIRECTION ( 'NONE',  ( 0.000000000000000000, 1.000000000000000000, 0.000000000000000000 ) ) ;
#13375=DIRECTION ( 'NONE',  ( 0.000000000000000000, -1.000000000000000000, 0.000000000000000000 ) ) ;
#13377=ORIENTED_EDGE ( 'NONE', *, *, #18721, .F. ) ;
#13382=ORIENTED_EDGE ( 'NONE', *, *, #21653, .T. ) ;
#13389=CIRCLE ( 'NONE', #6664, 0.3962400000000008138 ) ;
#13391=FACE_OUTER_BOUND ( 'NONE', #12365, .T. ) ;
#13397=DIRECTION ( 'NONE',  ( -1.000000000000000000, 0.000000000000000000, 0.000000000000000000 ) ) ;
#13400=VECTOR ( 'NONE', #8162, 1000.000000000000000 ) ;
#13402=VERTEX_POINT ( 'NONE', #3816 ) ;
#13403=CIRCLE ( 'NONE', #20121, 0.3962400000000008138 ) ;
#13405=CARTESIAN_POINT ( 'NONE',  ( 65.90927232300019512, 30.56064500000000095, -13.30734117861468135 ) ) ;
#13406=FACE_OUTER_BOUND ( 'NONE', #5641, .T. ) ;
#13410=CARTESIAN_POINT ( 'NONE',  ( 50.99913033092320092, 30.56064500000000095, -7.029081061492260751 ) ) ;
#13415=LINE ( 'NONE', #16517, #15287 ) ;
#13416=AXIS2_PLACEMENT_3D ( 'NONE', #6196, #14512, #11400 ) ;
#13429=CARTESIAN_POINT ( 'NONE',  ( 29.19635173153840313, 1.984375000000000000, -6.218966092919240296 ) ) ;
#13433=ORIENTED_EDGE ( 'NONE', *, *, #1432, .T. ) ;
#13435=DIRECTION ( 'NONE',  ( 0.2868778675745011220, 0.000000000000000000, 0.9579671649362033747 ) ) ;
#13437=EDGE_CURVE ( 'NONE', #18972, #8773, #8561, .T. ) ;
#13441=VECTOR ( 'NONE', #271, 1000.000000000000000 ) ;
#13446=DIRECTION ( 'NONE',  ( 0.000000000000000000, 1.000000000000000000, 0.000000000000000000 ) ) ;
#13461=DIRECTION ( 'NONE',  ( 0.000000000000000000, -1.000000000000000000, -6.251883472108000384E-09 ) ) ;
#13468=CARTESIAN_POINT ( 'NONE',  ( 1.954387715434429795, 23.81077936178774834, 10.71562499999999929 ) ) ;
#13474=AXIS2_PLACEMENT_3D ( 'NONE', #1286, #9571, #19632 ) ;
#13475=VERTEX_POINT ( 'NONE', #5461 ) ;
#13490=CARTESIAN_POINT ( 'NONE',  ( 28.97711086133420366, -42.42568807200000691, -10.71499000000000024 ) ) ;
#13501=LINE ( 'NONE', #20212, #3333 ) ;
#13507=CARTESIAN_POINT ( 'NONE',  ( 46.03750000000000142, 32.54502000000000095, -10.31874999999999964 ) ) ;
#13513=EDGE_CURVE ( 'NONE', #13567, #1356, #20602, .T. ) ;
#13525=CARTESIAN_POINT ( 'NONE',  ( -1.345424459097947834, 20.24316500000000119, 2.648158502653860324 ) ) ;
#13537=EDGE_CURVE ( 'NONE', #14260, #5609, #9103, .T. ) ;
#13551=ORIENTED_EDGE ( 'NONE', *, *, #11245, .F. ) ;
#13563=EDGE_CURVE ( 'NONE', #2020, #11999, #708, .T. ) ;
#13567=VERTEX_POINT ( 'NONE', #21267 ) ;
#13569=CYLINDRICAL_SURFACE ( 'NONE', #12343, 1.984375000000000000 ) ;
#13572=CARTESIAN_POINT ( 'NONE',  ( 66.03921914090641110, 1.984375000000000000, -11.33033647675950029 ) ) ;
#13573=ORIENTED_EDGE ( 'NONE', *, *, #17344, .T. ) ;
#13590=ORIENTED_EDGE ( 'NONE', *, *, #20425, .F. ) ;
#13599=ORIENTED_EDGE ( 'NONE', *, *, #14799, .F. ) ;
#13603=AXIS2_PLACEMENT_3D ( 'NONE', #12651, #10773, #4243 ) ;
#13612=ADVANCED_FACE ( 'NONE', ( #19053 ), #3930, .F. ) ;
#13617=FACE_BOUND ( 'NONE', #6218, .T. ) ;
#13625=LINE ( 'NONE', #16721, #8879 ) ;
#13629=DIRECTION ( 'NONE',  ( 1.000000000000000000, 0.000000000000000000, 0.000000000000000000 ) ) ;
#13635=VECTOR ( 'NONE', #133, 1000.000000000000000 ) ;
#13641=DIRECTION ( 'NONE',  ( -1.000000000000000000, 0.000000000000000000, 0.000000000000000000 ) ) ;
#13650=ORIENTED_EDGE ( 'NONE', *, *, #7092, .F. ) ;
#13655=SHAPE_DEFINITION_REPRESENTATION ( #11454, #21464 ) ;
#13656=CARTESIAN_POINT ( 'NONE',  ( -2.028188046367890074, 22.62314500000000095, 0.3682158094503220069 ) ) ;
#13658=DIRECTION ( 'NONE',  ( 1.000000000000000000, 0.000000000000000000, 0.000000000000000000 ) ) ;
#13688=EDGE_LOOP ( 'NONE', ( #16995, #5958, #19633, #13791 ) ) ;
#13689=ADVANCED_FACE ( 'NONE', ( #6009 ), #17528, .F. ) ;
#13691=DIRECTION ( 'NONE',  ( 0.000000000000000000, 1.000000000000000000, 0.000000000000000000 ) ) ;
#13693=FACE_OUTER_BOUND ( 'NONE', #16051, .T. ) ;
#13695=CARTESIAN_POINT ( 'NONE',  ( 1.786785375309217994, 8.953154907895765291, 10.71397434136291693 ) ) ;
#13698=CARTESIAN_POINT ( 'NONE',  ( -23.01875000000000071, 0.000000000000000000, -3.968750000000000000 ) ) ;
#13699=LINE ( 'NONE', #1958, #9491 ) ;
#13711=DIRECTION ( 'NONE',  ( -0.06191955310929838502, 0.000000000000000000, 0.9980811434661737147 ) ) ;
#13719=AXIS2_PLACEMENT_3D ( 'NONE', #8, #18582, #8736 ) ;
#13721=CARTESIAN_POINT ( 'NONE',  ( 65.47912282493159353, 0.000000000000000000, -13.30734117861468135 ) ) ;
#13738=ADVANCED_FACE ( 'NONE', ( #16523 ), #7892, .T. ) ;
#13739=VECTOR ( 'NONE', #6423, 1000.000000000000000 ) ;
#13745=VECTOR ( 'NONE', #19038, 1000.000000000000000 ) ;
#13754=CARTESIAN_POINT ( 'NONE',  ( 1.952969610814715207, 23.80837275291289856, 8.731249999999999289 ) ) ;
#13755=CARTESIAN_POINT ( 'NONE',  ( 66.03921914090641110, 0.000000000000000000, -11.33033647675950029 ) ) ;
#13759=CARTESIAN_POINT ( 'NONE',  ( 26.59062499999999929, 1.984057500000000251, 10.71562499999999929 ) ) ;
#13760=ADVANCED_FACE ( 'NONE', ( #9545 ), #14992, .T. ) ;
#13761=EDGE_LOOP ( 'NONE', ( #16771, #18641, #5072, #5381, #3914, #20619, #4748, #1395, #19339, #1040, #3139, #15348, #20733, #11716, #8685, #14621, #17734, #6127, #198, #632, #20977 ) ) ;
#13767=VERTEX_POINT ( 'NONE', #9859 ) ;
#13780=CIRCLE ( 'NONE', #4241, 3.175000000000000711 ) ;
#13790=CARTESIAN_POINT ( 'NONE',  ( 18.25624999999999787, 16.27314499999999953, 10.71562499999999929 ) ) ;
#13791=ORIENTED_EDGE ( 'NONE', *, *, #21666, .F. ) ;
#13795=VERTEX_POINT ( 'NONE', #21708 ) ;
#13817=CIRCLE ( 'NONE', #17684, 3.968750000000000000 ) ;
#13820=VERTEX_POINT ( 'NONE', #11438 ) ;
#13823=DIRECTION ( 'NONE',  ( 0.000000000000000000, 1.000000000000000000, 0.000000000000000000 ) ) ;
#13835=FACE_BOUND ( 'NONE', #15897, .T. ) ;
#13841=VECTOR ( 'NONE', #4553, 1000.000000000000000 ) ;
#13849=VERTEX_POINT ( 'NONE', #2931 ) ;
#13852=CARTESIAN_POINT ( 'NONE',  ( 65.64431122251959039, 0.000000000000000000, -11.29787305743958115 ) ) ;
#13854=VECTOR ( 'NONE', #2325, 1000.000000000000000 ) ;
#13857=CARTESIAN_POINT ( 'NONE',  ( 70.64340948846358970, 32.54502000000000095, -10.93409647675949969 ) ) ;
#13865=FACE_OUTER_BOUND ( 'NONE', #1215, .T. ) ;
#13868=CIRCLE ( 'NONE', #4325, 22.02656249999999005 ) ;
#13874=FACE_OUTER_BOUND ( 'NONE', #1187, .T. ) ;
#13884=LINE ( 'NONE', #1908, #13055 ) ;
#13929=DIRECTION ( 'NONE',  ( -0.6287118719681975554, 0.000000000000000000, -0.7776383362760898033 ) ) ;
#13948=ORIENTED_EDGE ( 'NONE', *, *, #5626, .F. ) ;
#13951=CARTESIAN_POINT ( 'NONE',  ( 8.309975510178299274, 0.1179876263055810032, 9.409168191377061063 ) ) ;
#13953=CARTESIAN_POINT ( 'NONE',  ( 66.03921914090641110, 32.54502000000000095, -10.93409647675949969 ) ) ;
#13956=VERTEX_POINT ( 'NONE', #8747 ) ;
#13958=AXIS2_PLACEMENT_3D ( 'NONE', #18479, #21694, #21795 ) ;
#13962=ORIENTED_EDGE ( 'NONE', *, *, #9543, .F. ) ;
#13974=LINE ( 'NONE', #10514, #6276 ) ;
#14005=ADVANCED_FACE ( 'NONE', ( #13874 ), #19473, .T. ) ;
#14009=FACE_OUTER_BOUND ( 'NONE', #1626, .T. ) ;
#14012=ORIENTED_EDGE ( 'NONE', *, *, #5270, .F. ) ;
#14021=ORIENTED_EDGE ( 'NONE', *, *, #943, .T. ) ;
#14022=CARTESIAN_POINT ( 'NONE',  ( 0.000000000000000000, 0.000000000000000000, 0.000000000000000000 ) ) ;
#14023=EDGE_CURVE ( 'NONE', #7714, #1266, #20796, .T. ) ;
#14026=LINE ( 'NONE', #622, #4740 ) ;
#14028=ORIENTED_EDGE ( 'NONE', *, *, #289, .T. ) ;
#14031=CARTESIAN_POINT ( 'NONE',  ( 67.79270099634359781, 1.984375000000000000, -13.76558698117381851 ) ) ;
#14033=DIRECTION ( 'NONE',  ( 0.000000000000000000, 1.000000000000000000, 0.000000000000000000 ) ) ;
#14038=DIRECTION ( 'NONE',  ( 1.000000000000000000, 0.000000000000000000, 0.000000000000000000 ) ) ;
#14048=ORIENTED_EDGE ( 'NONE', *, *, #7025, .F. ) ;
#14064=LINE ( 'NONE', #447, #20178 ) ;
#14068=LINE ( 'NONE', #3992, #13854 ) ;
#14082=CARTESIAN_POINT ( 'NONE',  ( -3.246390552019219999, 20.24316500000000119, 3.217431771123079987 ) ) ;
#14083=CARTESIAN_POINT ( 'NONE',  ( 46.03750000000000142, 0.000000000000000000, -10.31874999999999964 ) ) ;
#14086=DIRECTION ( 'NONE',  ( 0.000000000000000000, 0.000000000000000000, 1.000000000000000000 ) ) ;
#14091=DIRECTION ( 'NONE',  ( 0.000000000000000000, 1.000000000000000000, 0.000000000000000000 ) ) ;
#14095=ORIENTED_EDGE ( 'NONE', *, *, #7217, .T. ) ;
#14101=DIRECTION ( 'NONE',  ( -1.000000000000000000, 0.000000000000000000, 0.000000000000000000 ) ) ;
#14105=FACE_BOUND ( 'NONE', #731, .T. ) ;
#14112=DIRECTION ( 'NONE',  ( 0.000000000000000000, 1.000000000000000000, 0.000000000000000000 ) ) ;
#14116=DIRECTION ( 'NONE',  ( 0.000000000000000000, -1.000000000000000000, 0.000000000000000000 ) ) ;
#14119=DIRECTION ( 'NONE',  ( 0.000000000000000000, 1.000000000000000000, 0.000000000000000000 ) ) ;
#14133=AXIS2_PLACEMENT_3D ( 'NONE', #5144, #8568, #15227 ) ;
#14134=VERTEX_POINT ( 'NONE', #4120 ) ;
#14136=VECTOR ( 'NONE', #6641, 1000.000000000000000 ) ;
#14147=CARTESIAN_POINT ( 'NONE',  ( -160.2647810241784896, 30.16440499999999858, 8.335010000000000474 ) ) ;
#14150=LINE ( 'NONE', #7379, #5552 ) ;
#14159=VECTOR ( 'NONE', #2219, 1000.000000000000000 ) ;
#14162=VERTEX_POINT ( 'NONE', #17608 ) ;
#14164=VECTOR ( 'NONE', #14116, 1000.000000000000000 ) ;
#14171=CIRCLE ( 'NONE', #4618, 1.984374999999998890 ) ;
#14180=VECTOR ( 'NONE', #6923, 1000.000000000000000 ) ;
#14186=DIRECTION ( 'NONE',  ( 0.8334497143791951279, 0.000000000000000000, 0.5525953072558960066 ) ) ;
#14197=CARTESIAN_POINT ( 'NONE',  ( 1.954387715434429795, 23.41816500000000190, 6.745605000000000295 ) ) ;
#14201=CARTESIAN_POINT ( 'NONE',  ( 29.76562500000000000, 1.984375000000000000, -4.317999999999999616 ) ) ;
#14209=ORIENTED_EDGE ( 'NONE', *, *, #2487, .F. ) ;
#14216=VERTEX_POINT ( 'NONE', #14747 ) ;
#14218=PLANE ( 'NONE',  #13603 ) ;
#14220=ORIENTED_EDGE ( 'NONE', *, *, #16672, .F. ) ;
#14224=CARTESIAN_POINT ( 'NONE',  ( 65.90927232300019512, 30.56064500000000095, -13.30734117861468135 ) ) ;
#14228=DIRECTION ( 'NONE',  ( 0.1831666983862991482, 0.000000000000000000, -0.9830818687180954418 ) ) ;
#14238=DIRECTION ( 'NONE',  ( -1.000000000000000000, 0.000000000000000000, 0.000000000000000000 ) ) ;
#14241=CYLINDRICAL_SURFACE ( 'NONE', #14901, 3.175000000000000711 ) ;
#14243=DIRECTION ( 'NONE',  ( 0.000000000000000000, -1.000000000000000000, 0.000000000000000000 ) ) ;
#14248=EDGE_CURVE ( 'NONE', #3318, #19591, #11818, .T. ) ;
#14256=CIRCLE ( 'NONE', #7183, 0.3962400000000018130 ) ;
#14258=CARTESIAN_POINT ( 'NONE',  ( 29.36874999999999858, 9.921875000000000000, 8.731249999999999289 ) ) ;
#14260=VERTEX_POINT ( 'NONE', #11292 ) ;
#14263=DIRECTION ( 'NONE',  ( 0.000000000000000000, 1.000000000000000000, 0.000000000000000000 ) ) ;
#14264=ORIENTED_EDGE ( 'NONE', *, *, #14516, .T. ) ;
#14267=EDGE_LOOP ( 'NONE', ( #2988, #17328, #17346, #19897, #8712, #21641, #14264, #15580, #4667, #21746, #2137, #16877 ) ) ;
#14269=ADVANCED_FACE ( 'NONE', ( #9738 ), #7759, .F. ) ;
#14271=VECTOR ( 'NONE', #20787, 1000.000000000000000 ) ;
#14276=CIRCLE ( 'NONE', #14646, 0.3962399999999980382 ) ;
#14277=CARTESIAN_POINT ( 'NONE',  ( -1.880134707694870011, 20.24316500000000119, 7.779750394130780400 ) ) ;
#14291=EDGE_LOOP ( 'NONE', ( #20111, #12691, #1335, #10738 ) ) ;
#14300=EDGE_CURVE ( 'NONE', #2958, #21060, #1739, .T. ) ;
#14316=ORIENTED_EDGE ( 'NONE', *, *, #14670, .F. ) ;
#14320=CARTESIAN_POINT ( 'NONE',  ( 65.90927232300019512, 32.54502000000000095, -12.91110117861467899 ) ) ;
#14323=DIRECTION ( 'NONE',  ( 0.000000000000000000, 1.000000000000000000, 0.000000000000000000 ) ) ;
#14325=DIRECTION ( 'NONE',  ( 0.9579671649362032637, 0.000000000000000000, -0.2868778675745010664 ) ) ;
#14348=CARTESIAN_POINT ( 'NONE',  ( 1.538505192098342578, 9.095123825415061702, 8.691315493779447010 ) ) ;
#14360=LINE ( 'NONE', #10811, #3448 ) ;
#14382=CARTESIAN_POINT ( 'NONE',  ( -29.36874999999999858, 32.54502000000000095, -3.968750000000000000 ) ) ;
#14384=EDGE_CURVE ( 'NONE', #8281, #777, #9825, .T. ) ;
#14393=VERTEX_POINT ( 'NONE', #2179 ) ;
#14394=ORIENTED_EDGE ( 'NONE', *, *, #15751, .T. ) ;
#14395=DIRECTION ( 'NONE',  ( 0.000000000000000000, 1.000000000000000000, 0.000000000000000000 ) ) ;
#14396=EDGE_CURVE ( 'NONE', #17848, #18972, #13699, .T. ) ;
#14399=EDGE_CURVE ( 'NONE', #19126, #2537, #3629, .T. ) ;
#14413=EDGE_CURVE ( 'NONE', #6050, #138, #12250, .T. ) ;
#14419=CARTESIAN_POINT ( 'NONE',  ( 23.20826401227170166, 0.8126278217654899771, 10.33343709694782042 ) ) ;
#14423=FACE_BOUND ( 'NONE', #5471, .T. ) ;
#14427=DIRECTION ( 'NONE',  ( -0.7776383362760928009, 0.000000000000000000, 0.6287118719681937806 ) ) ;
#14434=PLANE ( 'NONE',  #11494 ) ;
#14435=EDGE_CURVE ( 'NONE', #10320, #16032, #15803, .T. ) ;
#14440=CARTESIAN_POINT ( 'NONE',  ( 29.36874999999999858, 22.62187499999999929, 8.731249999999999289 ) ) ;
#14448=ORIENTED_EDGE ( 'NONE', *, *, #15336, .F. ) ;
#14467=ORIENTED_EDGE ( 'NONE', *, *, #9373, .F. ) ;
#14468=CYLINDRICAL_SURFACE ( 'NONE', #5619, 0.3962399999999998146 ) ;
#14474=VECTOR ( 'NONE', #5990, 1000.000000000000000 ) ;
#14479=ORIENTED_EDGE ( 'NONE', *, *, #9889, .T. ) ;
#14482=DIRECTION ( 'NONE',  ( -0.2868778675745011220, 0.000000000000000000, -0.9579671649362033747 ) ) ;
#14486=EDGE_CURVE ( 'NONE', #11160, #16300, #17062, .T. ) ;
#14501=DIRECTION ( 'NONE',  ( -1.000000000000000000, 0.000000000000000000, 0.000000000000000000 ) ) ;
#14507=CYLINDRICAL_SURFACE ( 'NONE', #3658, 22.02656249999999361 ) ;
#14512=DIRECTION ( 'NONE',  ( 0.000000000000000000, -1.000000000000000000, 0.000000000000000000 ) ) ;
#14516=EDGE_CURVE ( 'NONE', #13956, #8026, #18709, .T. ) ;
#14518=DIRECTION ( 'NONE',  ( 0.000000000000000000, 0.000000000000000000, -1.000000000000000000 ) ) ;
#14521=CARTESIAN_POINT ( 'NONE',  ( 1.786968685778054455, 23.59452865405863875, 10.71398755195300900 ) ) ;
#14525=VERTEX_POINT ( 'NONE', #15322 ) ;
#14529=CIRCLE ( 'NONE', #8193, 1.984374999999998890 ) ;
#14530=CARTESIAN_POINT ( 'NONE',  ( 19.64159472326995015, 0.5582924111307500104, 10.11216594088294052 ) ) ;
#14533=CARTESIAN_POINT ( 'NONE',  ( -29.36874999999999858, 0.000000000000000000, 10.71562499999999929 ) ) ;
#14537=LINE ( 'NONE', #18056, #5444 ) ;
#14538=EDGE_CURVE ( 'NONE', #3944, #2217, #364, .T. ) ;
#14540=AXIS2_PLACEMENT_3D ( 'NONE', #14652, #1135, #16197 ) ;
#14541=CARTESIAN_POINT ( 'NONE',  ( -1.345424459097947834, 20.24316500000000119, 2.648158502653860324 ) ) ;
#14543=EDGE_CURVE ( 'NONE', #6593, #19545, #13884, .T. ) ;
#14544=CIRCLE ( 'NONE', #1455, 0.3962399999999998146 ) ;
#14545=DIRECTION ( 'NONE',  ( -0.2868778675745006224, -1.090993607693396258E-14, -0.9579671649362034858 ) ) ;
#14549=AXIS2_PLACEMENT_3D ( 'NONE', #12276, #20768, #9156 ) ;
#14562=PLANE ( 'NONE',  #9919 ) ;
#14565=AXIS2_PLACEMENT_3D ( 'NONE', #11289, #13191, #9833 ) ;
#14566=VECTOR ( 'NONE', #1212, 1000.000000000000000 ) ;
#14567=ORIENTED_EDGE ( 'NONE', *, *, #12188, .T. ) ;
#14568=LINE ( 'NONE', #9776, #8279 ) ;
#14571=CIRCLE ( 'NONE', #5008, 25.00312500000000426 ) ;
#14580=VECTOR ( 'NONE', #4082, 1000.000000000000000 ) ;
#14593=ORIENTED_EDGE ( 'NONE', *, *, #2790, .T. ) ;
#14596=ORIENTED_EDGE ( 'NONE', *, *, #21779, .T. ) ;
#14597=EDGE_CURVE ( 'NONE', #14993, #18115, #2357, .T. ) ;
#14604=CARTESIAN_POINT ( 'NONE',  ( 49.09065990372640442, 30.56064500000000095, -26.70549589918839928 ) ) ;
#14612=DIRECTION ( 'NONE',  ( 0.000000000000000000, -1.000000000000000000, 0.000000000000000000 ) ) ;
#14621=ORIENTED_EDGE ( 'NONE', *, *, #19905, .F. ) ;
#14622=ORIENTED_EDGE ( 'NONE', *, *, #10605, .F. ) ;
#14625=VECTOR ( 'NONE', #20072, 1000.000000000000227 ) ;
#14628=EDGE_CURVE ( 'NONE', #11489, #5739, #18317, .T. ) ;
#14645=ORIENTED_EDGE ( 'NONE', *, *, #15539, .F. ) ;
#14646=AXIS2_PLACEMENT_3D ( 'NONE', #8289, #20312, #1752 ) ;
#14652=CARTESIAN_POINT ( 'NONE',  ( 67.40134256979101224, 32.54502000000000095, -13.70358117861468017 ) ) ;
#14654=EDGE_CURVE ( 'NONE', #21761, #14134, #9088, .T. ) ;
#14659=CARTESIAN_POINT ( 'NONE',  ( 70.64340948846358970, 74.97070807199999365, -10.53785647675949910 ) ) ;
#14664=DIRECTION ( 'NONE',  ( 0.000000000000000000, 1.000000000000000000, 0.000000000000000000 ) ) ;
#14667=ORIENTED_EDGE ( 'NONE', *, *, #1561, .F. ) ;
#14670=EDGE_CURVE ( 'NONE', #12461, #14393, #13389, .T. ) ;
#14681=CARTESIAN_POINT ( 'NONE',  ( 49.16323787629939801, 1.984375000000000000, -27.09503225884920141 ) ) ;
#14682=ORIENTED_EDGE ( 'NONE', *, *, #9698, .T. ) ;
#14683=ADVANCED_FACE ( 'NONE', ( #14423, #7662 ), #15865, .T. ) ;
#14684=CARTESIAN_POINT ( 'NONE',  ( -29.36874999999999858, 1.984375000000000000, 8.335010000000000474 ) ) ;
#14693=DIRECTION ( 'NONE',  ( 0.000000000000000000, 1.000000000000000000, 0.000000000000000000 ) ) ;
#14695=LINE ( 'NONE', #2838, #825 ) ;
#14698=EDGE_LOOP ( 'NONE', ( #1801, #17665, #4844, #12207 ) ) ;
#14699=EDGE_CURVE ( 'NONE', #19591, #18990, #1378, .T. ) ;
#14704=LINE ( 'NONE', #16775, #20860 ) ;
#14724=ORIENTED_EDGE ( 'NONE', *, *, #10354, .F. ) ;
#14730=DIRECTION ( 'NONE',  ( 0.000000000000000000, 0.000000000000000000, 1.000000000000000000 ) ) ;
#14739=DIRECTION ( 'NONE',  ( 1.000000000000000000, 0.000000000000000000, 0.000000000000000000 ) ) ;
#14740=CIRCLE ( 'NONE', #13331, 9.524999999999998579 ) ;
#14746=ORIENTED_EDGE ( 'NONE', *, *, #7539, .F. ) ;
#14747=CARTESIAN_POINT ( 'NONE',  ( -23.81250000000000000, 16.27314499999999953, 8.731249999999999289 ) ) ;
#14757=FILL_AREA_STYLE ('',( #16408 ) ) ;
#14763=CARTESIAN_POINT ( 'NONE',  ( -29.36874999999999858, 0.000000000000000000, -3.968750000000000000 ) ) ;
#14766=CARTESIAN_POINT ( 'NONE',  ( 71.03305177384599745, 0.000000000000000000, -10.93409647675949969 ) ) ;
#14781=ORIENTED_EDGE ( 'NONE', *, *, #7706, .F. ) ;
#14782=CARTESIAN_POINT ( 'NONE',  ( 28.97711086133420366, 1.984375000000000000, -10.31874999999999964 ) ) ;
#14795=DIRECTION ( 'NONE',  ( -0.9966381950048638361, 0.000000000000000000, 0.08192867786951606168 ) ) ;
#14796=EDGE_CURVE ( 'NONE', #966, #14216, #17733, .T. ) ;
#14799=EDGE_CURVE ( 'NONE', #8773, #2714, #2082, .T. ) ;
#14808=EDGE_LOOP ( 'NONE', ( #14724, #12591, #19872, #19415 ) ) ;
#14813=EDGE_CURVE ( 'NONE', #6814, #1714, #5622, .T. ) ;
#14819=VERTEX_POINT ( 'NONE', #16724 ) ;
#14821=DIRECTION ( 'NONE',  ( 0.000000000000000000, -1.000000000000000000, 6.254384957144000359E-09 ) ) ;
#14825=LINE ( 'NONE', #4752, #13400 ) ;
#14833=CARTESIAN_POINT ( 'NONE',  ( 26.59062499999999929, 1.984057500000000251, 10.71562499999999929 ) ) ;
#14846=DIRECTION ( 'NONE',  ( -1.000000000000000000, 0.000000000000000000, 0.000000000000000000 ) ) ;
#14850=CARTESIAN_POINT ( 'NONE',  ( -21.43124999999999858, 30.56064500000000095, -4.860316984116058095E-16 ) ) ;
#14866=AXIS2_PLACEMENT_3D ( 'NONE', #581, #5660, #354 ) ;
#14875=DIRECTION ( 'NONE',  ( 0.000000000000000000, 1.000000000000000000, 0.000000000000000000 ) ) ;
#14876=VECTOR ( 'NONE', #4760, 1000.000000000000000 ) ;
#14894=VECTOR ( 'NONE', #10658, 1000.000000000000000 ) ;
#14895=ADVANCED_FACE ( 'NONE', ( #11745 ), #4881, .F. ) ;
#14896=AXIS2_PLACEMENT_3D ( 'NONE', #11450, #19834, #8011 ) ;
#14901=AXIS2_PLACEMENT_3D ( 'NONE', #10793, #2273, #2386 ) ;
#14902=DIRECTION ( 'NONE',  ( 0.000000000000000000, 1.000000000000000000, 0.000000000000000000 ) ) ;
#14904=EDGE_CURVE ( 'NONE', #9456, #7901, #1453, .T. ) ;
#14906=CARTESIAN_POINT ( 'NONE',  ( -17.46249999999999858, 0.000000000000000000, 0.000000000000000000 ) ) ;
#14915=CARTESIAN_POINT ( 'NONE',  ( 29.76562500000000000, 32.54502000000000095, -4.317999999999999616 ) ) ;
#14919=EDGE_CURVE ( 'NONE', #5923, #3431, #8084, .T. ) ;
#14925=VERTEX_POINT ( 'NONE', #13405 ) ;
#14959=DIRECTION ( 'NONE',  ( 0.000000000000000000, 1.000000000000000000, 0.000000000000000000 ) ) ;
#14968=DIRECTION ( 'NONE',  ( -0.5733392046337749681, 0.8193181045417647912, 0.000000000000000000 ) ) ;
#14973=ADVANCED_FACE ( 'NONE', ( #16305 ), #1140, .T. ) ;
#14977=CARTESIAN_POINT ( 'NONE',  ( 30.33489826846160398, 30.56064500000000095, -2.417033907079745525 ) ) ;
#14980=ORIENTED_EDGE ( 'NONE', *, *, #20702, .F. ) ;
#14982=AXIS2_PLACEMENT_3D ( 'NONE', #4843, #11581, #8684 ) ;
#14992=CYLINDRICAL_SURFACE ( 'NONE', #7445, 25.00312499999999361 ) ;
#14993=VERTEX_POINT ( 'NONE', #6324 ) ;
#14996=DIRECTION ( 'NONE',  ( 0.000000000000000000, 0.000000000000000000, 1.000000000000000000 ) ) ;
#15014=AXIS2_PLACEMENT_3D ( 'NONE', #19695, #9748, #14427 ) ;
#15017=ORIENTED_EDGE ( 'NONE', *, *, #319, .F. ) ;
#15020=DIRECTION ( 'NONE',  ( 0.000000000000000000, 0.000000000000000000, -1.000000000000000000 ) ) ;
#15026=CARTESIAN_POINT ( 'NONE',  ( -1.345424459097947834, 12.30439499999999953, 2.648158502653860324 ) ) ;
#15037=CARTESIAN_POINT ( 'NONE',  ( -23.01875000000000071, 30.56064500000000095, -10.31874999999999964 ) ) ;
#15038=FACE_OUTER_BOUND ( 'NONE', #418, .T. ) ;
#15047=EDGE_CURVE ( 'NONE', #11999, #6050, #18481, .T. ) ;
#15067=CYLINDRICAL_SURFACE ( 'NONE', #6049, 25.00312499999999361 ) ;
#15072=EDGE_CURVE ( 'NONE', #7901, #17335, #20885, .T. ) ;
#15078=DIRECTION ( 'NONE',  ( 1.000000000000000000, 0.000000000000000000, 0.000000000000000000 ) ) ;
#15081=DIRECTION ( 'NONE',  ( 0.000000000000000000, 1.000000000000000000, 0.000000000000000000 ) ) ;
#15089=DIRECTION ( 'NONE',  ( -0.9579671649362034858, 0.000000000000000000, 0.2868778675745011220 ) ) ;
#15094=ORIENTED_EDGE ( 'NONE', *, *, #7913, .T. ) ;
#15104=ORIENTED_EDGE ( 'NONE', *, *, #7193, .T. ) ;
#15110=ORIENTED_EDGE ( 'NONE', *, *, #1891, .T. ) ;
#15114=DIRECTION ( 'NONE',  ( 0.000000000000000000, 1.000000000000000000, 0.000000000000000000 ) ) ;
#15120=ORIENTED_EDGE ( 'NONE', *, *, #8143, .T. ) ;
#15123=EDGE_LOOP ( 'NONE', ( #16153, #18793, #1954, #4946 ) ) ;
#15134=ORIENTED_EDGE ( 'NONE', *, *, #6248, .T. ) ;
#15137=DIRECTION ( 'NONE',  ( 1.000000000000000000, 0.000000000000000000, 0.000000000000000000 ) ) ;
#15147=ORIENTED_EDGE ( 'NONE', *, *, #705, .T. ) ;
#15152=ORIENTED_EDGE ( 'NONE', *, *, #17760, .T. ) ;
#15154=ORIENTED_EDGE ( 'NONE', *, *, #9623, .F. ) ;
#15163=DIRECTION ( 'NONE',  ( -0.9579671649362033747, 0.000000000000000000, 0.2868778675745011220 ) ) ;
#15166=CARTESIAN_POINT ( 'NONE',  ( 65.90927232300019512, 32.54502000000000095, -13.30734117861468135 ) ) ;
#15193=DIRECTION ( 'NONE',  ( 0.000000000000000000, 1.000000000000000000, 0.000000000000000000 ) ) ;
#15196=ORIENTED_EDGE ( 'NONE', *, *, #14300, .F. ) ;
#15199=VERTEX_POINT ( 'NONE', #16171 ) ;
#15201=CARTESIAN_POINT ( 'NONE',  ( -23.01875000000000071, 0.000000000000000000, -3.968750000000000000 ) ) ;
#15206=LINE ( 'NONE', #21821, #17353 ) ;
#15211=ORIENTED_EDGE ( 'NONE', *, *, #15611, .F. ) ;
#15217=AXIS2_PLACEMENT_3D ( 'NONE', #20094, #16485, #1319 ) ;
#15227=DIRECTION ( 'NONE',  ( 1.000000000000000000, 0.000000000000000000, 0.000000000000000000 ) ) ;
#15231=ORIENTED_EDGE ( 'NONE', *, *, #7195, .F. ) ;
#15243=ORIENTED_EDGE ( 'NONE', *, *, #7613, .F. ) ;
#15253=B_SPLINE_CURVE_WITH_KNOTS ( 'NONE', 3,
 ( #9304, #7755, #14521, #1331, #13080, #16078, #908, #11081 ),
 .UNSPECIFIED., .F., .F.,
 ( 4, 2, 2, 4 ),
 ( 0.000000000000000000, 0.4999999999999966693, 0.7499999999999983347, 1.000000000000000000 ),
 .UNSPECIFIED. ) ;
#15256=DIRECTION ( 'NONE',  ( 0.9876802608827760510, 0.000000000000000000, -0.1564854698127960131 ) ) ;
#15261=VERTEX_POINT ( 'NONE', #6851 ) ;
#15262=CIRCLE ( 'NONE', #5351, 9.524999999999998579 ) ;
#15267=ORIENTED_EDGE ( 'NONE', *, *, #11245, .T. ) ;
#15269=FACE_OUTER_BOUND ( 'NONE', #9441, .T. ) ;
#15278=CARTESIAN_POINT ( 'NONE',  ( 1.268730000000000135, 9.129395000000000593, 8.609509071587499562 ) ) ;
#15279=DIRECTION ( 'NONE',  ( 0.9876802608827758290, 0.000000000000000000, -0.1564854698127972066 ) ) ;
#15287=VECTOR ( 'NONE', #5001, 1000.000000000000000 ) ;
#15293=ORIENTED_EDGE ( 'NONE', *, *, #735, .F. ) ;
#15297=AXIS2_PLACEMENT_3D ( 'NONE', #17907, #14612, #17808 ) ;
#15306=DIRECTION ( 'NONE',  ( 0.2868778675745010664, 0.000000000000000000, 0.9579671649362032637 ) ) ;
#15310=DIRECTION ( 'NONE',  ( -0.9966381950048638361, 0.000000000000000000, 0.08192867786951606168 ) ) ;
#15313=ORIENTED_EDGE ( 'NONE', *, *, #15345, .T. ) ;
#15317=AXIS2_PLACEMENT_3D ( 'NONE', #16202, #9850, #1027 ) ;
#15319=EDGE_CURVE ( 'NONE', #18275, #5609, #4596, .T. ) ;
#15322=CARTESIAN_POINT ( 'NONE',  ( 6.585898268469219552, 0.000000000000000000, 4.694966092919240275 ) ) ;
#15324=ORIENTED_EDGE ( 'NONE', *, *, #8819, .F. ) ;
#15336=EDGE_CURVE ( 'NONE', #2932, #6593, #7417, .T. ) ;
#15341=ORIENTED_EDGE ( 'NONE', *, *, #11108, .T. ) ;
#15342=ORIENTED_EDGE ( 'NONE', *, *, #19537, .T. ) ;
#15345=EDGE_CURVE ( 'NONE', #11015, #16300, #9173, .T. ) ;
#15348=ORIENTED_EDGE ( 'NONE', *, *, #14813, .F. ) ;
#15352=ORIENTED_EDGE ( 'NONE', *, *, #7195, .T. ) ;
#15353=ADVANCED_FACE ( 'NONE', ( #12555 ), #4138, .T. ) ;
#15358=LINE ( 'NONE', #8364, #6441 ) ;
#15361=VECTOR ( 'NONE', #2027, 1000.000000000000000 ) ;
#15367=EDGE_CURVE ( 'NONE', #7181, #7389, #19811, .T. ) ;
#15381=PLANE ( 'NONE',  #21223 ) ;
#15382=VERTEX_POINT ( 'NONE', #12885 ) ;
#15386=ORIENTED_EDGE ( 'NONE', *, *, #2047, .F. ) ;
#15401=EDGE_LOOP ( 'NONE', ( #9234, #13962, #19099, #10355 ) ) ;
#15416=ADVANCED_FACE ( 'NONE', ( #8640 ), #10186, .F. ) ;
#15420=DIRECTION ( 'NONE',  ( -0.9966381950048638361, 0.000000000000000000, 0.08192867786951606168 ) ) ;
#15441=CARTESIAN_POINT ( 'NONE',  ( 2.063750000000000195, 8.334374999999999645, 10.71562499999999929 ) ) ;
#15450=CARTESIAN_POINT ( 'NONE',  ( 30.33489826846160398, 1.984375000000000000, -2.417033907079745525 ) ) ;
#15457=EDGE_LOOP ( 'NONE', ( #10487, #15479, #70, #5370, #11477, #13599 ) ) ;
#15466=EDGE_CURVE ( 'NONE', #1261, #7354, #2829, .T. ) ;
#15468=CARTESIAN_POINT ( 'NONE',  ( 67.40134256979101224, 32.54502000000000095, -13.30734117861468135 ) ) ;
#15479=ORIENTED_EDGE ( 'NONE', *, *, #7880, .F. ) ;
#15486=DIRECTION ( 'NONE',  ( 0.000000000000000000, 0.000000000000000000, -1.000000000000000000 ) ) ;
#15490=CARTESIAN_POINT ( 'NONE',  ( 65.64431122251959039, 30.56064500000000095, -11.29787305743958115 ) ) ;
#15493=VECTOR ( 'NONE', #6642, 1000.000000000000000 ) ;
#15503=ORIENTED_EDGE ( 'NONE', *, *, #13563, .F. ) ;
#15512=LINE ( 'NONE', #13857, #15493 ) ;
#15521=DIRECTION ( 'NONE',  ( -0.9579671649362034858, 0.000000000000000000, 0.2868778675745010109 ) ) ;
#15531=AXIS2_PLACEMENT_3D ( 'NONE', #4988, #4785, #15078 ) ;
#15536=CARTESIAN_POINT ( 'NONE',  ( 29.76562500000000000, 1.984375000000000000, -4.317999999999999616 ) ) ;
#15539=EDGE_CURVE ( 'NONE', #19746, #7932, #19899, .T. ) ;
#15542=VERTEX_POINT ( 'NONE', #16385 ) ;
#15563=ORIENTED_EDGE ( 'NONE', *, *, #20540, .T. ) ;
#15564=EDGE_CURVE ( 'NONE', #15989, #15924, #17929, .T. ) ;
#15567=STYLED_ITEM ( 'NONE', ( #16508 ), #6635 ) ;
#15573=DIRECTION ( 'NONE',  ( -0.2868778675745008999, 0.000000000000000000, -0.9579671649362034858 ) ) ;
#15580=ORIENTED_EDGE ( 'NONE', *, *, #3589, .F. ) ;
#15581=ORIENTED_EDGE ( 'NONE', *, *, #12494, .F. ) ;
#15590=EDGE_CURVE ( 'NONE', #2743, #7573, #12159, .T. ) ;
#15591=ORIENTED_EDGE ( 'NONE', *, *, #1644, .F. ) ;
#15592=EDGE_CURVE ( 'NONE', #15542, #1856, #4394, .T. ) ;
#15611=EDGE_CURVE ( 'NONE', #15199, #10916, #13501, .T. ) ;
#15618=EDGE_LOOP ( 'NONE', ( #4984, #11234, #21011, #15110 ) ) ;
#15631=CIRCLE ( 'NONE', #9249, 19.05000000000000071 ) ;
#15634=EDGE_CURVE ( 'NONE', #7573, #15261, #3648, .T. ) ;
#15640=AXIS2_PLACEMENT_3D ( 'NONE', #13053, #19656, #6180 ) ;
#15647=ADVANCED_FACE ( 'NONE', ( #11933 ), #3532, .T. ) ;
#15649=VECTOR ( 'NONE', #3258, 1000.000000000000227 ) ;
#15656=ORIENTED_EDGE ( 'NONE', *, *, #8002, .F. ) ;
#15668=DIRECTION ( 'NONE',  ( 0.000000000000000000, 1.000000000000000000, 0.000000000000000000 ) ) ;
#15671=EDGE_CURVE ( 'NONE', #12065, #18576, #1713, .T. ) ;
#15673=EDGE_LOOP ( 'NONE', ( #2609, #16661, #3199, #4508 ) ) ;
#15677=DIRECTION ( 'NONE',  ( 0.000000000000000000, 0.000000000000000000, 1.000000000000000000 ) ) ;
#15681=CYLINDRICAL_SURFACE ( 'NONE', #5685, 2.381250000000001421 ) ;
#15686=CYLINDRICAL_SURFACE ( 'NONE', #13232, 0.3962400000000010358 ) ;
#15687=AXIS2_PLACEMENT_3D ( 'NONE', #1142, #1249, #6221 ) ;
#15695=DIRECTION ( 'NONE',  ( 0.000000000000000000, -1.000000000000000000, 0.000000000000000000 ) ) ;
#15716=CARTESIAN_POINT ( 'NONE',  ( 14.35012762246612006, 0.3010510652611559923, 9.783890749713020085 ) ) ;
#15718=CARTESIAN_POINT ( 'NONE',  ( 1.782353389576713409, 23.59070174808080012, 8.727807302940615131 ) ) ;
#15722=DIRECTION ( 'NONE',  ( 1.000000000000000000, 0.000000000000000000, 0.000000000000000000 ) ) ;
#15730=ORIENTED_EDGE ( 'NONE', *, *, #17924, .T. ) ;
#15736=ORIENTED_EDGE ( 'NONE', *, *, #19522, .T. ) ;
#15737=CARTESIAN_POINT ( 'NONE',  ( 71.03963378001139972, 32.54502000000000095, -10.54138470677948014 ) ) ;
#15740=CARTESIAN_POINT ( 'NONE',  ( 31.75000000000000000, 32.54502000000000095, -4.317999999999999616 ) ) ;
#15744=ADVANCED_FACE ( 'NONE', ( #5401 ), #17465, .T. ) ;
#15746=AXIS2_PLACEMENT_3D ( 'NONE', #20077, #4944, #11696 ) ;
#15751=EDGE_CURVE ( 'NONE', #10775, #9189, #1893, .T. ) ;
#15752=CARTESIAN_POINT ( 'NONE',  ( -12.30312499999999964, 1.984375000000000000, -2.268784209304649746 ) ) ;
#15768=FACE_BOUND ( 'NONE', #9132, .T. ) ;
#15789=CARTESIAN_POINT ( 'NONE',  ( 1.952969610814715207, 8.739187247087119914, 8.731249999999999289 ) ) ;
#15803=LINE ( 'NONE', #5601, #19727 ) ;
#15804=DIRECTION ( 'NONE',  ( 0.000000000000000000, 1.000000000000000000, 0.000000000000000000 ) ) ;
#15810=ORIENTED_EDGE ( 'NONE', *, *, #10074, .T. ) ;
#15817=EDGE_CURVE ( 'NONE', #16263, #6310, #18120, .T. ) ;
#15821=DIRECTION ( 'NONE',  ( 0.000000000000000000, 0.000000000000000000, -1.000000000000000000 ) ) ;
#15824=AXIS2_PLACEMENT_3D ( 'NONE', #1648, #3004, #15163 ) ;
#15829=DIRECTION ( 'NONE',  ( -0.9579671649362033747, 0.000000000000000000, 0.2868778675745011220 ) ) ;
#15844=VECTOR ( 'NONE', #8634, 1000.000000000000000 ) ;
#15854=DIRECTION ( 'NONE',  ( 0.000000000000000000, -1.000000000000000000, 0.000000000000000000 ) ) ;
#15857=CARTESIAN_POINT ( 'NONE',  ( 21.03437500000000071, 1.984375000000000000, 5.159374999999999822 ) ) ;
#15865=PLANE ( 'NONE',  #21850 ) ;
#15868=ORIENTED_EDGE ( 'NONE', *, *, #15972, .F. ) ;
#15877=CARTESIAN_POINT ( 'NONE',  ( 46.03750000000000142, 1.984375000000000000, -10.31874999999999964 ) ) ;
#15884=CARTESIAN_POINT ( 'NONE',  ( 54.11611804786240043, 32.54502000000000095, -30.58983753981140197 ) ) ;
#15890=ORIENTED_EDGE ( 'NONE', *, *, #20190, .F. ) ;
#15897=EDGE_LOOP ( 'NONE', ( #4184, #15937 ) ) ;
#15899=DIRECTION ( 'NONE',  ( -0.1831666983862943188, 0.000000000000000000, 0.9830818687180962190 ) ) ;
#15901=VECTOR ( 'NONE', #937, 1000.000000000000000 ) ;
#15904=CARTESIAN_POINT ( 'NONE',  ( 2.063750000000000195, 30.16440499999999858, 8.335010000000000474 ) ) ;
#15907=DIRECTION ( 'NONE',  ( 1.000000000000000000, 0.000000000000000000, 0.000000000000000000 ) ) ;
#15908=EDGE_CURVE ( 'NONE', #19333, #1356, #7942, .T. ) ;
#15920=ORIENTED_EDGE ( 'NONE', *, *, #15367, .F. ) ;
#15924=VERTEX_POINT ( 'NONE', #19400 ) ;
#15927=CIRCLE ( 'NONE', #2484, 25.00312500000000426 ) ;
#15931=AXIS2_PLACEMENT_3D ( 'NONE', #14906, #21622, #18098 ) ;
#15933=LINE ( 'NONE', #7292, #12150 ) ;
#15934=DIRECTION ( 'NONE',  ( 0.000000000000000000, 0.000000000000000000, 1.000000000000000000 ) ) ;
#15937=ORIENTED_EDGE ( 'NONE', *, *, #14628, .T. ) ;
#15940=CARTESIAN_POINT ( 'NONE',  ( -20.63749999999999929, 16.27314499999999953, 8.731249999999999289 ) ) ;
#15944=VERTEX_POINT ( 'NONE', #17769 ) ;
#15957=AXIS2_PLACEMENT_3D ( 'NONE', #13656, #6574, #6787 ) ;
#15958=CIRCLE ( 'NONE', #13474, 2.381250000000001421 ) ;
#15967=LINE ( 'NONE', #19258, #19474 ) ;
#15972=EDGE_CURVE ( 'NONE', #20891, #11142, #14026, .T. ) ;
#15983=VERTEX_POINT ( 'NONE', #7692 ) ;
#15987=AXIS2_PLACEMENT_3D ( 'NONE', #9812, #18231, #16259 ) ;
#15989=VERTEX_POINT ( 'NONE', #20837 ) ;
#15992=LINE ( 'NONE', #5895, #7852 ) ;
#15998=EDGE_CURVE ( 'NONE', #9031, #7389, #852, .T. ) ;
#16004=ORIENTED_EDGE ( 'NONE', *, *, #7432, .T. ) ;
#16012=LINE ( 'NONE', #840, #8064 ) ;
#16019=ADVANCED_FACE ( 'NONE', ( #10569 ), #15686, .F. ) ;
#16022=DIRECTION ( 'NONE',  ( 0.000000000000000000, 0.000000000000000000, -1.000000000000000000 ) ) ;
#16029=ORIENTED_EDGE ( 'NONE', *, *, #12764, .F. ) ;
#16032=VERTEX_POINT ( 'NONE', #14684 ) ;
#16036=AXIS2_PLACEMENT_3D ( 'NONE', #17158, #5423, #9178 ) ;
#16040=EDGE_CURVE ( 'NONE', #2429, #6204, #7797, .T. ) ;
#16041=DIRECTION ( 'NONE',  ( 0.000000000000000000, 1.000000000000000000, 0.000000000000000000 ) ) ;
#16046=ORIENTED_EDGE ( 'NONE', *, *, #19326, .F. ) ;
#16049=DIRECTION ( 'NONE',  ( 0.000000000000000000, 0.000000000000000000, -1.000000000000000000 ) ) ;
#16050=CARTESIAN_POINT ( 'NONE',  ( 71.04062499999999147, 32.54502000000000095, -10.31874999999999964 ) ) ;
#16051=EDGE_LOOP ( 'NONE', ( #13015, #19878, #7731, #12108 ) ) ;
#16060=LINE ( 'NONE', #7740, #6029 ) ;
#16063=DIRECTION ( 'NONE',  ( 0.000000000000000000, 1.000000000000000000, 0.000000000000000000 ) ) ;
#16068=EDGE_CURVE ( 'NONE', #6310, #7268, #14568, .T. ) ;
#16071=AXIS2_PLACEMENT_3D ( 'NONE', #13410, #15081, #13312 ) ;
#16078=CARTESIAN_POINT ( 'NONE',  ( 1.403477590199228464, 23.42690089012609178, 10.67779458928513314 ) ) ;
#16081=ORIENTED_EDGE ( 'NONE', *, *, #20425, .T. ) ;
#16085=CARTESIAN_POINT ( 'NONE',  ( 29.36900889036359885, 1.958445551117574901, 10.71563714734171846 ) ) ;
#16087=CARTESIAN_POINT ( 'NONE',  ( -23.81250000000000000, 16.27314499999999953, 8.731249999999999289 ) ) ;
#16088=EDGE_LOOP ( 'NONE', ( #16759, #13254, #21606, #19546, #9896, #6913, #326 ) ) ;
#16089=LINE ( 'NONE', #5888, #4985 ) ;
#16113=VERTEX_POINT ( 'NONE', #9876 ) ;
#16124=DIRECTION ( 'NONE',  ( -0.9579671649362032637, 0.000000000000000000, 0.2868778675745010664 ) ) ;
#16139=ORIENTED_EDGE ( 'NONE', *, *, #5898, .F. ) ;
#16153=ORIENTED_EDGE ( 'NONE', *, *, #9625, .F. ) ;
#16165=DIRECTION ( 'NONE',  ( 0.000000000000000000, 1.000000000000000000, 0.000000000000000000 ) ) ;
#16170=FACE_OUTER_BOUND ( 'NONE', #19297, .T. ) ;
#16171=CARTESIAN_POINT ( 'NONE',  ( 6.585898268469219552, 32.54502000000000095, 4.694966092919240275 ) ) ;
#16178=LINE ( 'NONE', #1004, #20563 ) ;
#16184=CARTESIAN_POINT ( 'NONE',  ( -12.30312499999999964, 30.16440499999999858, 8.335010000000000474 ) ) ;
#16188=LINE ( 'NONE', #19369, #7473 ) ;
#16191=EDGE_CURVE ( 'NONE', #14525, #12822, #20703, .T. ) ;
#16197=DIRECTION ( 'NONE',  ( 0.000000000000000000, 0.000000000000000000, 1.000000000000000000 ) ) ;
#16202=CARTESIAN_POINT ( 'NONE',  ( 21.03437500000000071, 30.56064500000000095, 5.159374999999999822 ) ) ;
#16204=LINE ( 'NONE', #12886, #18809 ) ;
#16206=CARTESIAN_POINT ( 'NONE',  ( 6.016625000000000334, 30.56064500000000095, 2.794000000000000039 ) ) ;
#16208=CARTESIAN_POINT ( 'NONE',  ( 26.59062499999999929, 5.953125000000000000, 8.731249999999999289 ) ) ;
#16212=VERTEX_POINT ( 'NONE', #5558 ) ;
#16219=LINE ( 'NONE', #12460, #3232 ) ;
#16220=ORIENTED_EDGE ( 'NONE', *, *, #14384, .F. ) ;
#16223=AXIS2_PLACEMENT_3D ( 'NONE', #1694, #3474, #7121 ) ;
#16245=ORIENTED_EDGE ( 'NONE', *, *, #21811, .F. ) ;
#16246=ORIENTED_EDGE ( 'NONE', *, *, #5082, .F. ) ;
#16257=DIRECTION ( 'NONE',  ( 0.000000000000000000, -1.000000000000000000, 0.000000000000000000 ) ) ;
#16258=LINE ( 'NONE', #6280, #10295 ) ;
#16259=DIRECTION ( 'NONE',  ( 0.3850029901312932989, 0.000000000000000000, -0.9229153252546862252 ) ) ;
#16263=VERTEX_POINT ( 'NONE', #12315 ) ;
#16264=EDGE_CURVE ( 'NONE', #11872, #20613, #17828, .T. ) ;
#16269=DIRECTION ( 'NONE',  ( -0.9999999998269335499, -1.860465115957061339E-05, 0.000000000000000000 ) ) ;
#16272=ORIENTED_EDGE ( 'NONE', *, *, #4694, .F. ) ;
#16283=VECTOR ( 'NONE', #3605, 1000.000000000000000 ) ;
#16300=VERTEX_POINT ( 'NONE', #12436 ) ;
#16301=CARTESIAN_POINT ( 'NONE',  ( -2.607150795738780058, 32.54502000000000095, 8.731885000000000119 ) ) ;
#16305=FACE_OUTER_BOUND ( 'NONE', #9797, .T. ) ;
#16307=ADVANCED_FACE ( 'NONE', ( #4132, #19042, #15768, #14105, #8876 ), #14218, .F. ) ;
#16315=DIRECTION ( 'NONE',  ( 1.000000000000000000, 0.000000000000000000, 0.000000000000000000 ) ) ;
#16316=ORIENTED_EDGE ( 'NONE', *, *, #12926, .F. ) ;
#16323=CARTESIAN_POINT ( 'NONE',  ( 54.36523883999320361, 0.000000000000000000, -30.28170612544299800 ) ) ;
#16331=AXIS2_PLACEMENT_3D ( 'NONE', #13698, #12025, #3628 ) ;
#16340=ORIENTED_EDGE ( 'NONE', *, *, #6650, .F. ) ;
#16344=ORIENTED_EDGE ( 'NONE', *, *, #316, .T. ) ;
#16345=CARTESIAN_POINT ( 'NONE',  ( 54.36523883999320361, 74.97070807199999365, -30.28170612544299800 ) ) ;
#16352=ORIENTED_EDGE ( 'NONE', *, *, #12494, .T. ) ;
#16357=AXIS2_PLACEMENT_3D ( 'NONE', #14197, #796, #15521 ) ;
#16364=DIRECTION ( 'NONE',  ( -0.1727088819286940469, 0.000000000000000000, 0.9849729144006653669 ) ) ;
#16369=VECTOR ( 'NONE', #8972, 1000.000000000000227 ) ;
#16376=EDGE_LOOP ( 'NONE', ( #15581, #18656, #5139, #10998 ) ) ;
#16378=CARTESIAN_POINT ( 'NONE',  ( 55.56250000000000000, 1.984375000000000000, -10.31874999999999964 ) ) ;
#16385=CARTESIAN_POINT ( 'NONE',  ( 66.87634738983680904, 30.56064500000000095, 3.497859541731999755 ) ) ;
#16393=DIRECTION ( 'NONE',  ( 0.000000000000000000, 0.000000000000000000, 1.000000000000000000 ) ) ;
#16394=DIRECTION ( 'NONE',  ( 0.2868778675745004558, 0.000000000000000000, 0.9579671649362035968 ) ) ;
#16405=DIRECTION ( 'NONE',  ( 0.000000000000000000, 1.000000000000000000, 0.000000000000000000 ) ) ;
#16407=ADVANCED_FACE ( 'NONE', ( #1344 ), #17849, .F. ) ;
#16408=FILL_AREA_STYLE_COLOUR ( '', #20821 ) ;
#16415=ADVANCED_FACE ( 'NONE', ( #19489 ), #21580, .T. ) ;
#16417=AXIS2_PLACEMENT_3D ( 'NONE', #18272, #4893, #14545 ) ;
#16420=DIRECTION ( 'NONE',  ( 0.000000000000000000, 1.000000000000000000, 0.000000000000000000 ) ) ;
#16426=CARTESIAN_POINT ( 'NONE',  ( 29.19635173153840313, 0.000000000000000000, -6.218966092919240296 ) ) ;
#16429=ORIENTED_EDGE ( 'NONE', *, *, #13437, .F. ) ;
#16438=DIRECTION ( 'NONE',  ( 0.000000000000000000, 1.000000000000000000, 0.000000000000000000 ) ) ;
#16447=CARTESIAN_POINT ( 'NONE',  ( 29.37324403177899868, 30.56064500000000095, -10.70578951775076071 ) ) ;
#16450=ORIENTED_EDGE ( 'NONE', *, *, #8047, .F. ) ;
#16457=CARTESIAN_POINT ( 'NONE',  ( 2.063750000000000195, 30.56064500000000095, 8.335010000000000474 ) ) ;
#16458=ORIENTED_EDGE ( 'NONE', *, *, #14023, .F. ) ;
#16464=CIRCLE ( 'NONE', #13283, 0.3962399999999988154 ) ;
#16465=EDGE_LOOP ( 'NONE', ( #1641, #3776, #8786, #4532 ) ) ;
#16475=DIRECTION ( 'NONE',  ( 1.000000000000000000, 0.000000000000000000, 0.000000000000000000 ) ) ;
#16485=DIRECTION ( 'NONE',  ( 0.000000000000000000, 1.000000000000000000, 0.000000000000000000 ) ) ;
#16506=CARTESIAN_POINT ( 'NONE',  ( 28.97711086133420366, 30.56064500000000095, -10.31874999999999964 ) ) ;
#16508=PRESENTATION_STYLE_ASSIGNMENT (( #4680 ) ) ;
#16517=CARTESIAN_POINT ( 'NONE',  ( -160.2647810241784896, 30.56064500000000095, 10.71562489836746046 ) ) ;
#16519=CYLINDRICAL_SURFACE ( 'NONE', #1260, 0.3962400000000008138 ) ;
#16523=FACE_OUTER_BOUND ( 'NONE', #14808, .T. ) ;
#16529=EDGE_CURVE ( 'NONE', #15944, #21849, #14537, .T. ) ;
#16531=CARTESIAN_POINT ( 'NONE',  ( 0.05261182704408059324, 9.129395000000000593, 7.316601101023040066 ) ) ;
#16536=VERTEX_POINT ( 'NONE', #21256 ) ;
#16537=LINE ( 'NONE', #6021, #4290 ) ;
#16540=ORIENTED_EDGE ( 'NONE', *, *, #15611, .T. ) ;
#16573=EDGE_CURVE ( 'NONE', #9687, #15542, #18171, .T. ) ;
#16574=CYLINDRICAL_SURFACE ( 'NONE', #857, 2.381250000000001421 ) ;
#16579=ORIENTED_EDGE ( 'NONE', *, *, #1543, .F. ) ;
#16590=CARTESIAN_POINT ( 'NONE',  ( 2.063750000000000195, 24.21318500000000284, 8.731249999999999289 ) ) ;
#16598=ADVANCED_FACE ( 'NONE', ( #1776 ), #6645, .T. ) ;
#16600=CIRCLE ( 'NONE', #17355, 1.984374999999998890 ) ;
#16603=FACE_OUTER_BOUND ( 'NONE', #2327, .T. ) ;
#16616=DIRECTION ( 'NONE',  ( 0.000000000000000000, -1.000000000000000000, 0.000000000000000000 ) ) ;
#16625=DIRECTION ( 'NONE',  ( -0.2868778675745010664, 0.000000000000000000, -0.9579671649362032637 ) ) ;
#16633=FACE_OUTER_BOUND ( 'NONE', #11359, .T. ) ;
#16635=DIRECTION ( 'NONE',  ( 0.000000000000000000, 1.000000000000000000, 0.000000000000000000 ) ) ;
#16639=FACE_OUTER_BOUND ( 'NONE', #5261, .T. ) ;
#16643=AXIS2_PLACEMENT_3D ( 'NONE', #15857, #12305, #12424 ) ;
#16648=CARTESIAN_POINT ( 'NONE',  ( -4.157227781567939928, 22.62314500000000095, 0.1758860224507720060 ) ) ;
#16652=ADVANCED_FACE ( 'NONE', ( #4992, #20015 ), #125, .T. ) ;
#16656=ORIENTED_EDGE ( 'NONE', *, *, #14300, .T. ) ;
#16661=ORIENTED_EDGE ( 'NONE', *, *, #11972, .T. ) ;
#16663=DIRECTION ( 'NONE',  ( 0.000000000000000000, 1.000000000000000000, 0.000000000000000000 ) ) ;
#16665=FACE_OUTER_BOUND ( 'NONE', #5585, .T. ) ;
#16668=ORIENTED_EDGE ( 'NONE', *, *, #16898, .F. ) ;
#16672=EDGE_CURVE ( 'NONE', #21532, #18768, #6876, .T. ) ;
#16678=EDGE_CURVE ( 'NONE', #8026, #14393, #8636, .T. ) ;
#16680=DIRECTION ( 'NONE',  ( 0.000000000000000000, -1.000000000000000000, 0.000000000000000000 ) ) ;
#16681=LINE ( 'NONE', #1522, #10389 ) ;
#16686=EDGE_LOOP ( 'NONE', ( #628, #19441, #4368, #10026 ) ) ;
#16687=DIRECTION ( 'NONE',  ( 0.000000000000000000, -1.000000000000000000, 0.000000000000000000 ) ) ;
#16689=DIRECTION ( 'NONE',  ( 0.000000000000000000, 0.000000000000000000, -1.000000000000000000 ) ) ;
#16690=DIRECTION ( 'NONE',  ( 0.000000000000000000, 1.000000000000000000, 0.000000000000000000 ) ) ;
#16698=LINE ( 'NONE', #14833, #20131 ) ;
#16706=AXIS2_PLACEMENT_3D ( 'NONE', #9184, #7753, #12417 ) ;
#16708=DIRECTION ( 'NONE',  ( 0.000000000000000000, 1.000000000000000000, 0.000000000000000000 ) ) ;
#16715=CARTESIAN_POINT ( 'NONE',  ( -29.36874999999999858, 1.984375000000000000, -3.968750000000000000 ) ) ;
#16721=CARTESIAN_POINT ( 'NONE',  ( 29.36874999999999858, 22.62187499999999929, 8.731249999999999289 ) ) ;
#16724=CARTESIAN_POINT ( 'NONE',  ( 67.40134256979101224, 1.984375000000000000, -13.30734117861468135 ) ) ;
#16726=EDGE_CURVE ( 'NONE', #4424, #19957, #16729, .T. ) ;
#16729=LINE ( 'NONE', #11631, #4010 ) ;
#16736=CARTESIAN_POINT ( 'NONE',  ( 49.16323787629939801, 30.56064500000000095, -27.09503225884920141 ) ) ;
#16738=CARTESIAN_POINT ( 'NONE',  ( 29.19635173153840313, 30.56064500000000095, -6.218966092919240296 ) ) ;
#16739=DIRECTION ( 'NONE',  ( 0.000000000000000000, 0.000000000000000000, 1.000000000000000000 ) ) ;
#16754=CYLINDRICAL_SURFACE ( 'NONE', #17706, 19.05000000000000426 ) ;
#16759=ORIENTED_EDGE ( 'NONE', *, *, #1108, .T. ) ;
#16771=ORIENTED_EDGE ( 'NONE', *, *, #9625, .T. ) ;
#16773=DIRECTION ( 'NONE',  ( 1.000000000000000000, 0.000000000000000000, 0.000000000000000000 ) ) ;
#16775=CARTESIAN_POINT ( 'NONE',  ( 67.40134256979101224, 1.984375000000000000, -13.30734117861468135 ) ) ;
#16779=ADVANCED_FACE ( 'NONE', ( #17043 ), #3123, .F. ) ;
#16780=VERTEX_POINT ( 'NONE', #8311 ) ;
#16789=CARTESIAN_POINT ( 'NONE',  ( -17.46249999999999858, 0.000000000000000000, 0.000000000000000000 ) ) ;
#16790=FACE_OUTER_BOUND ( 'NONE', #11361, .T. ) ;
#16791=FACE_BOUND ( 'NONE', #8959, .T. ) ;
#16797=DIRECTION ( 'NONE',  ( 0.000000000000000000, 1.000000000000000000, 0.000000000000000000 ) ) ;
#16800=CARTESIAN_POINT ( 'NONE',  ( 18.65312499999999929, 32.54502000000000095, 5.159374999999999822 ) ) ;
#16804=ADVANCED_FACE ( 'NONE', ( #10415 ), #572, .F. ) ;
#16809=PLANE ( 'NONE',  #15824 ) ;
#16812=CARTESIAN_POINT ( 'NONE',  ( 67.79270099634359781, 32.54502000000000095, -13.76558698117381851 ) ) ;
#16817=ORIENTED_EDGE ( 'NONE', *, *, #14799, .T. ) ;
#16825=LINE ( 'NONE', #8087, #5287 ) ;
#16826=CARTESIAN_POINT ( 'NONE',  ( 26.59062499999999929, 30.56064500000000095, 8.731249999999999289 ) ) ;
#16831=LINE ( 'NONE', #21701, #19168 ) ;
#16846=DIRECTION ( 'NONE',  ( 1.000000000000000000, 0.000000000000000000, 0.000000000000000000 ) ) ;
#16877=ORIENTED_EDGE ( 'NONE', *, *, #7880, .T. ) ;
#16880=DIRECTION ( 'NONE',  ( 0.000000000000000000, 1.000000000000000000, 0.000000000000000000 ) ) ;
#16890=CARTESIAN_POINT ( 'NONE',  ( -20.63749999999999929, 16.27314499999999953, 10.71562499999999929 ) ) ;
#16895=( GEOMETRIC_REPRESENTATION_CONTEXT ( 3 ) GLOBAL_UNCERTAINTY_ASSIGNED_CONTEXT ( ( #17631 ) ) GLOBAL_UNIT_ASSIGNED_CONTEXT ( ( #6573, #18193, #21607 ) ) REPRESENTATION_CONTEXT ( 'NONE', 'WORKASPACE' ) );
#16898=EDGE_CURVE ( 'NONE', #14819, #17008, #21291, .T. ) ;
#16900=CARTESIAN_POINT ( 'NONE',  ( 49.16323787629939801, 0.000000000000000000, -27.09503225884920141 ) ) ;
#16907=EDGE_CURVE ( 'NONE', #7705, #17225, #21019, .T. ) ;
#16920=ORIENTED_EDGE ( 'NONE', *, *, #7913, .F. ) ;
#16934=VECTOR ( 'NONE', #4901, 1000.000000000000227 ) ;
#16943=LINE ( 'NONE', #13759, #21767 ) ;
#16944=FACE_BOUND ( 'NONE', #10401, .T. ) ;
#16946=VECTOR ( 'NONE', #7877, 1000.000000000000000 ) ;
#16949=CARTESIAN_POINT ( 'NONE',  ( 31.75000000000000000, 30.56064500000000095, -4.317999999999999616 ) ) ;
#16959=EDGE_CURVE ( 'NONE', #1266, #11872, #4331, .T. ) ;
#16969=ORIENTED_EDGE ( 'NONE', *, *, #12926, .T. ) ;
#16980=CARTESIAN_POINT ( 'NONE',  ( 71.03305177384599745, 0.000000000000000000, -10.93409647675949969 ) ) ;
#16983=AXIS2_PLACEMENT_3D ( 'NONE', #15026, #11358, #20062 ) ;
#16986=CARTESIAN_POINT ( 'NONE',  ( 21.03437500000000071, 0.000000000000000000, 5.159374999999999822 ) ) ;
#16990=DIRECTION ( 'NONE',  ( 0.000000000000000000, -1.000000000000000000, 0.000000000000000000 ) ) ;
#16993=VECTOR ( 'NONE', #7429, 999.9999999999998863 ) ;
#16995=ORIENTED_EDGE ( 'NONE', *, *, #2974, .T. ) ;
#17002=ORIENTED_EDGE ( 'NONE', *, *, #5327, .F. ) ;
#17008=VERTEX_POINT ( 'NONE', #17709 ) ;
#17015=VECTOR ( 'NONE', #16689, 1000.000000000000000 ) ;
#17022=CARTESIAN_POINT ( 'NONE',  ( 1.268730000000000135, 9.129395000000000593, 10.65596716962832069 ) ) ;
#17026=CARTESIAN_POINT ( 'NONE',  ( 55.56250000000000000, 0.000000000000000000, -10.31874999999999964 ) ) ;
#17027=DIRECTION ( 'NONE',  ( 0.000000000000000000, 1.000000000000000000, 0.000000000000000000 ) ) ;
#17032=CARTESIAN_POINT ( 'NONE',  ( -2.028188046367890074, 23.41816500000000190, 0.3682158094503220069 ) ) ;
#17036=AXIS2_PLACEMENT_3D ( 'NONE', #15201, #10099, #16846 ) ;
#17037=LINE ( 'NONE', #15737, #9533 ) ;
#17043=FACE_OUTER_BOUND ( 'NONE', #10912, .T. ) ;
#17048=DIRECTION ( 'NONE',  ( 1.000000000000000000, 0.000000000000000000, 0.000000000000000000 ) ) ;
#17062=LINE ( 'NONE', #1798, #11263 ) ;
#17064=PLANE ( 'NONE',  #20442 ) ;
#17076=VECTOR ( 'NONE', #10930, 1000.000000000000000 ) ;
#17096=FACE_OUTER_BOUND ( 'NONE', #14291, .T. ) ;
#17105=DIRECTION ( 'NONE',  ( 0.9980811434661737147, 0.000000000000000000, 0.06191955310929838502 ) ) ;
#17107=VECTOR ( 'NONE', #20573, 1000.000000000000114 ) ;
#17112=ORIENTED_EDGE ( 'NONE', *, *, #16068, .T. ) ;
#17113=FACE_OUTER_BOUND ( 'NONE', #17782, .T. ) ;
#17115=PLANE ( 'NONE',  #19431 ) ;
#17116=ADVANCED_FACE ( 'NONE', ( #16170 ), #14507, .T. ) ;
#17119=ORIENTED_EDGE ( 'NONE', *, *, #5327, .T. ) ;
#17120=ADVANCED_FACE ( 'NONE', ( #21640 ), #6501, .T. ) ;
#17135=DIRECTION ( 'NONE',  ( 0.000000000000000000, 1.000000000000000000, 0.000000000000000000 ) ) ;
#17158=CARTESIAN_POINT ( 'NONE',  ( 29.36874999999999858, 22.62187499999999929, 8.731249999999999289 ) ) ;
#17160=CARTESIAN_POINT ( 'NONE',  ( 46.03750000000000142, 0.000000000000000000, -10.31874999999999964 ) ) ;
#17165=LINE ( 'NONE', #18, #13635 ) ;
#17174=DIRECTION ( 'NONE',  ( 0.2868778675745004558, 0.000000000000000000, 0.9579671649362035968 ) ) ;
#17181=ORIENTED_EDGE ( 'NONE', *, *, #7225, .T. ) ;
#17195=DIRECTION ( 'NONE',  ( 0.000000000000000000, 1.000000000000000000, 0.000000000000000000 ) ) ;
#17202=CIRCLE ( 'NONE', #21794, 9.524999999999998579 ) ;
#17204=ORIENTED_EDGE ( 'NONE', *, *, #17650, .F. ) ;
#17206=EDGE_CURVE ( 'NONE', #6814, #3875, #5253, .T. ) ;
#17225=VERTEX_POINT ( 'NONE', #13468 ) ;
#17230=ORIENTED_EDGE ( 'NONE', *, *, #13040, .T. ) ;
#17241=DIRECTION ( 'NONE',  ( 0.000000000000000000, 1.000000000000000000, 0.000000000000000000 ) ) ;
#17269=CIRCLE ( 'NONE', #8433, 3.175000000000000711 ) ;
#17287=EDGE_CURVE ( 'NONE', #15983, #6204, #20282, .T. ) ;
#17299=AXIS2_PLACEMENT_3D ( 'NONE', #8008, #1161, #11219 ) ;
#17303=ORIENTED_EDGE ( 'NONE', *, *, #16529, .F. ) ;
#17318=DIRECTION ( 'NONE',  ( 0.000000000000000000, 1.000000000000000000, 0.000000000000000000 ) ) ;
#17319=VERTEX_POINT ( 'NONE', #5371 ) ;
#17323=CARTESIAN_POINT ( 'NONE',  ( 29.76562500000000000, 32.54502000000000095, -4.317999999999999616 ) ) ;
#17328=ORIENTED_EDGE ( 'NONE', *, *, #7217, .F. ) ;
#17331=DIRECTION ( 'NONE',  ( -1.000000000000000000, 0.000000000000000000, 0.000000000000000000 ) ) ;
#17332=DIRECTION ( 'NONE',  ( 1.000000000000000000, 0.000000000000000000, 0.000000000000000000 ) ) ;
#17335=VERTEX_POINT ( 'NONE', #10133 ) ;
#17336=ORIENTED_EDGE ( 'NONE', *, *, #6781, .T. ) ;
#17344=EDGE_CURVE ( 'NONE', #13849, #12892, #11330, .T. ) ;
#17345=ORIENTED_EDGE ( 'NONE', *, *, #764, .T. ) ;
#17346=ORIENTED_EDGE ( 'NONE', *, *, #12382, .T. ) ;
#17353=VECTOR ( 'NONE', #4817, 1000.000000000000000 ) ;
#17355=AXIS2_PLACEMENT_3D ( 'NONE', #15536, #10435, #17174 ) ;
#17361=DIRECTION ( 'NONE',  ( -0.000000000000000000, 1.000000000000000000, 0.000000000000000000 ) ) ;
#17367=VERTEX_POINT ( 'NONE', #21513 ) ;
#17370=DIRECTION ( 'NONE',  ( 1.000000000000000000, 0.000000000000000000, 0.000000000000000000 ) ) ;
#17373=ADVANCED_FACE ( 'NONE', ( #860 ), #14468, .T. ) ;
#17376=DIRECTION ( 'NONE',  ( 0.000000000000000000, -1.000000000000000000, 0.000000000000000000 ) ) ;
#17381=DIRECTION ( 'NONE',  ( 0.000000000000000000, 1.000000000000000000, 0.000000000000000000 ) ) ;
#17383=AXIS2_PLACEMENT_3D ( 'NONE', #1417, #4750, #18328 ) ;
#17384=VECTOR ( 'NONE', #7061, 999.9999999999998863 ) ;
#17394=FACE_OUTER_BOUND ( 'NONE', #11829, .T. ) ;
#17399=CARTESIAN_POINT ( 'NONE',  ( -1.848761088705630051, 9.129395000000000593, 7.884515871828260636 ) ) ;
#17405=EDGE_CURVE ( 'NONE', #18990, #12688, #17988, .T. ) ;
#17419=CIRCLE ( 'NONE', #5752, 0.3962399999999980382 ) ;
#17421=DIRECTION ( 'NONE',  ( -0.8192319205190408127, 0.5734623443633278805, 0.000000000000000000 ) ) ;
#17430=CARTESIAN_POINT ( 'NONE',  ( 29.76562500000000000, 32.54502000000000095, -4.317999999999999616 ) ) ;
#17433=ORIENTED_EDGE ( 'NONE', *, *, #14248, .T. ) ;
#17435=PLANE ( 'NONE',  #21459 ) ;
#17436=EDGE_LOOP ( 'NONE', ( #4490, #15154, #12846, #4322 ) ) ;
#17444=CARTESIAN_POINT ( 'NONE',  ( 1.538729348984987588, 9.085401985160794780, 10.69440411747507724 ) ) ;
#17445=ORIENTED_EDGE ( 'NONE', *, *, #12328, .F. ) ;
#17455=ORIENTED_EDGE ( 'NONE', *, *, #12764, .T. ) ;
#17459=ORIENTED_EDGE ( 'NONE', *, *, #3615, .F. ) ;
#17461=EDGE_LOOP ( 'NONE', ( #16540, #15730, #18337, #7811 ) ) ;
#17463=CARTESIAN_POINT ( 'NONE',  ( 16.72089543368710096, 0.4026526316987140142, 9.930969856814060748 ) ) ;
#17464=LINE ( 'NONE', #10723, #6143 ) ;
#17465=CYLINDRICAL_SURFACE ( 'NONE', #10386, 0.3962399999999975386 ) ;
#17473=FACE_OUTER_BOUND ( 'NONE', #3724, .T. ) ;
#17477=ADVANCED_FACE ( 'NONE', ( #6808 ), #13569, .F. ) ;
#17495=CIRCLE ( 'NONE', #3024, 0.3962399999999988154 ) ;
#17496=DIRECTION ( 'NONE',  ( 0.000000000000000000, 0.000000000000000000, -1.000000000000000000 ) ) ;
#17502=DIRECTION ( 'NONE',  ( 0.000000000000000000, 1.000000000000000000, 0.000000000000000000 ) ) ;
#17506=DIRECTION ( 'NONE',  ( 0.000000000000000000, 0.000000000000000000, -1.000000000000000000 ) ) ;
#17515=CARTESIAN_POINT ( 'NONE',  ( 71.03963378001139972, 1.984375000000000000, -10.54138470677948014 ) ) ;
#17523=ADVANCED_FACE ( 'NONE', ( #3492 ), #9792, .F. ) ;
#17524=CARTESIAN_POINT ( 'NONE',  ( 70.64340948846358970, 0.000000000000000000, -10.53785647675949910 ) ) ;
#17528=CYLINDRICAL_SURFACE ( 'NONE', #19428, 0.7950200000000000600 ) ;
#17539=ORIENTED_EDGE ( 'NONE', *, *, #6248, .F. ) ;
#17557=CARTESIAN_POINT ( 'NONE',  ( 54.36523883999320361, 1.984375000000000000, -30.28170612544299800 ) ) ;
#17567=ORIENTED_EDGE ( 'NONE', *, *, #10354, .T. ) ;
#17571=DIRECTION ( 'NONE',  ( 0.9876802608827760510, 0.000000000000000000, -0.1564854698127960131 ) ) ;
#17572=CARTESIAN_POINT ( 'NONE',  ( 29.36874999999999858, 22.62187499999999929, 10.71562499999999929 ) ) ;
#17580=CARTESIAN_POINT ( 'NONE',  ( 36.51250000000000284, 32.54502000000000095, -10.31875000000000142 ) ) ;
#17583=EDGE_CURVE ( 'NONE', #6627, #2217, #4835, .T. ) ;
#17592=CARTESIAN_POINT ( 'NONE',  ( -29.36874999999999858, 30.56128000000000000, 10.71562499999999929 ) ) ;
#17604=DIRECTION ( 'NONE',  ( 0.2868778675745004558, 0.000000000000000000, 0.9579671649362035968 ) ) ;
#17605=CARTESIAN_POINT ( 'NONE',  ( 46.03750000000000142, 0.000000000000000000, -10.31874999999999964 ) ) ;
#17608=CARTESIAN_POINT ( 'NONE',  ( 49.09065990372640442, 32.54502000000000095, -26.70549589918839928 ) ) ;
#17616=ORIENTED_EDGE ( 'NONE', *, *, #9786, .F. ) ;
#17631=UNCERTAINTY_MEASURE_WITH_UNIT (LENGTH_MEASURE( 1.000000000000000082E-05 ), #6573, 'distance_accuracy_value', 'NONE');
#17643=EDGE_LOOP ( 'NONE', ( #13222, #21628, #18987, #12477, #6525, #1420, #17567, #5701, #18447, #4605, #21812, #21447, #3051, #15341, #18296, #15147, #15591, #15313, #1831, #10274, #5952, #6806, #9636, #19735, #4207, #20967, #7184 ) ) ;
#17644=DIRECTION ( 'NONE',  ( 1.000000000000000000, 0.000000000000000000, 0.000000000000000000 ) ) ;
#17650=EDGE_CURVE ( 'NONE', #19545, #12822, #2383, .T. ) ;
#17655=DIRECTION ( 'NONE',  ( 0.000000000000000000, 1.000000000000000000, 0.000000000000000000 ) ) ;
#17658=CARTESIAN_POINT ( 'NONE',  ( -23.81250000000000000, 16.27314499999999953, 10.71562499999999929 ) ) ;
#17663=LINE ( 'NONE', #2512, #9145 ) ;
#17664=DIRECTION ( 'NONE',  ( 0.000000000000000000, 1.000000000000000000, 0.000000000000000000 ) ) ;
#17665=ORIENTED_EDGE ( 'NONE', *, *, #13537, .T. ) ;
#17674=VECTOR ( 'NONE', #11956, 1000.000000000000000 ) ;
#17682=CARTESIAN_POINT ( 'NONE',  ( 1.880866719892425376, 23.68649982446676816, 8.731249999999999289 ) ) ;
#17684=AXIS2_PLACEMENT_3D ( 'NONE', #18769, #313, #10895 ) ;
#17685=ORIENTED_EDGE ( 'NONE', *, *, #5107, .T. ) ;
#17691=DIRECTION ( 'NONE',  ( 0.000000000000000000, 1.000000000000000000, 0.000000000000000000 ) ) ;
#17692=ORIENTED_EDGE ( 'NONE', *, *, #21352, .T. ) ;
#17695=CARTESIAN_POINT ( 'NONE',  ( -2.028188046367890074, 23.41816500000000190, 0.3682158094503220069 ) ) ;
#17706=AXIS2_PLACEMENT_3D ( 'NONE', #18288, #8659, #6998 ) ;
#17709=CARTESIAN_POINT ( 'NONE',  ( 67.79270099634359781, 1.984375000000000000, -13.76558698117381851 ) ) ;
#17719=FACE_OUTER_BOUND ( 'NONE', #1256, .T. ) ;
#17728=CARTESIAN_POINT ( 'NONE',  ( 24.28501924911759957, 0.9100045512280500182, 10.40023748037497953 ) ) ;
#17729=EDGE_CURVE ( 'NONE', #4043, #19124, #13403, .T. ) ;
#17730=AXIS2_PLACEMENT_3D ( 'NONE', #20219, #18248, #11940 ) ;
#17733=LINE ( 'NONE', #16087, #14474 ) ;
#17734=ORIENTED_EDGE ( 'NONE', *, *, #17897, .F. ) ;
#17743=DIRECTION ( 'NONE',  ( 0.000000000000000000, -1.000000000000000000, 0.000000000000000000 ) ) ;
#17744=AXIS2_PLACEMENT_3D ( 'NONE', #6065, #12836, #8476 ) ;
#17753=CIRCLE ( 'NONE', #19142, 0.7950200000000005041 ) ;
#17757=CARTESIAN_POINT ( 'NONE',  ( -21.43124999999999858, 1.984375000000000000, -4.860316984116058095E-16 ) ) ;
#17760=EDGE_CURVE ( 'NONE', #1714, #11015, #391, .T. ) ;
#17767=ORIENTED_EDGE ( 'NONE', *, *, #2336, .T. ) ;
#17769=CARTESIAN_POINT ( 'NONE',  ( -29.36874999999999858, 0.000000000000000000, -3.968750000000000000 ) ) ;
#17773=CIRCLE ( 'NONE', #94, 19.05000000000001137 ) ;
#17782=EDGE_LOOP ( 'NONE', ( #11062, #5831, #2542, #14209 ) ) ;
#17783=ORIENTED_EDGE ( 'NONE', *, *, #15047, .F. ) ;
#17794=ORIENTED_EDGE ( 'NONE', *, *, #11808, .T. ) ;
#17795=DIRECTION ( 'NONE',  ( 0.000000000000000000, 1.000000000000000000, 0.000000000000000000 ) ) ;
#17799=DIRECTION ( 'NONE',  ( 1.000000000000000000, 0.000000000000000000, 0.000000000000000000 ) ) ;
#17808=DIRECTION ( 'NONE',  ( 1.000000000000000000, 0.000000000000000000, 0.000000000000000000 ) ) ;
#17809=CARTESIAN_POINT ( 'NONE',  ( -21.43124999999999858, 32.54502000000000095, -4.860316984116058095E-16 ) ) ;
#17828=CIRCLE ( 'NONE', #2641, 0.7950200000000005041 ) ;
#17837=FACE_BOUND ( 'NONE', #9126, .T. ) ;
#17839=AXIS2_PLACEMENT_3D ( 'NONE', #4307, #7514, #15934 ) ;
#17844=CARTESIAN_POINT ( 'NONE',  ( 29.21834112936799954, 1.789188963192005044, 10.70629397521275905 ) ) ;
#17846=CARTESIAN_POINT ( 'NONE',  ( 26.59062499999999929, 30.16440499999999858, 8.335010000000000474 ) ) ;
#17848=VERTEX_POINT ( 'NONE', #833 ) ;
#17849=CYLINDRICAL_SURFACE ( 'NONE', #518, 2.381250000000001421 ) ;
#17852=CARTESIAN_POINT ( 'NONE',  ( 65.90927232300019512, 0.000000000000000000, -12.91110117861467899 ) ) ;
#17853=DIRECTION ( 'NONE',  ( -0.9579671649362032637, 0.000000000000000000, 0.2868778675745010664 ) ) ;
#17862=VERTEX_POINT ( 'NONE', #17757 ) ;
#17869=ORIENTED_EDGE ( 'NONE', *, *, #1704, .F. ) ;
#17883=CARTESIAN_POINT ( 'NONE',  ( -13.49374999999999858, 30.56064500000000095, 0.000000000000000000 ) ) ;
#17889=DIRECTION ( 'NONE',  ( 1.000000000000000000, 0.000000000000000000, 0.000000000000000000 ) ) ;
#17890=ORIENTED_EDGE ( 'NONE', *, *, #14597, .T. ) ;
#17895=VECTOR ( 'NONE', #11058, 1000.000000000000000 ) ;
#17897=EDGE_CURVE ( 'NONE', #2743, #17319, #21056, .T. ) ;
#17899=CARTESIAN_POINT ( 'NONE',  ( 18.25624999999999787, 16.27314499999999953, 8.731249999999999289 ) ) ;
#17901=CARTESIAN_POINT ( 'NONE',  ( -21.43124999999999858, 0.000000000000000000, -4.860316984116058095E-16 ) ) ;
#17903=ORIENTED_EDGE ( 'NONE', *, *, #5876, .T. ) ;
#17907=CARTESIAN_POINT ( 'NONE',  ( 46.03750000000000142, 32.54502000000000095, -10.31874999999999964 ) ) ;
#17908=EDGE_CURVE ( 'NONE', #16300, #6460, #21512, .T. ) ;
#17924=EDGE_CURVE ( 'NONE', #10916, #6719, #4375, .T. ) ;
#17925=EDGE_CURVE ( 'NONE', #13767, #13956, #10890, .T. ) ;
#17929=LINE ( 'NONE', #6088, #20971 ) ;
#17933=ORIENTED_EDGE ( 'NONE', *, *, #7404, .T. ) ;
#17941=ORIENTED_EDGE ( 'NONE', *, *, #20867, .T. ) ;
#17945=CARTESIAN_POINT ( 'NONE',  ( 66.03921914090641110, 0.000000000000000000, -10.93409647675949969 ) ) ;
#17961=DIRECTION ( 'NONE',  ( 1.000000000000000000, 0.000000000000000000, 0.000000000000000000 ) ) ;
#17962=EDGE_CURVE ( 'NONE', #14925, #3318, #9148, .T. ) ;
#17978=ORIENTED_EDGE ( 'NONE', *, *, #10600, .T. ) ;
#17984=ORIENTED_EDGE ( 'NONE', *, *, #11479, .F. ) ;
#17988=LINE ( 'NONE', #958, #11671 ) ;
#18001=CARTESIAN_POINT ( 'NONE',  ( 29.19635173153840313, 32.54502000000000095, -6.218966092919240296 ) ) ;
#18003=CARTESIAN_POINT ( 'NONE',  ( 65.90927232300019512, 1.984375000000000000, -12.91110117861467899 ) ) ;
#18008=CARTESIAN_POINT ( 'NONE',  ( -23.01875000000000071, 1.984375000000000000, -10.31874999999999964 ) ) ;
#18015=MECHANICAL_DESIGN_GEOMETRIC_PRESENTATION_REPRESENTATION('',(#15567),#1058);
#18028=VECTOR ( 'NONE', #3201, 1000.000000000000227 ) ;
#18048=CARTESIAN_POINT ( 'NONE',  ( 27.23577668703720178, 1.270868477333907842, 10.58329832977197960 ) ) ;
#18054=AXIS2_PLACEMENT_3D ( 'NONE', #9691, #21846, #18420 ) ;
#18055=CARTESIAN_POINT ( 'NONE',  ( 54.11611804786240043, 1.984375000000000000, -30.58983753981140197 ) ) ;
#18056=CARTESIAN_POINT ( 'NONE',  ( -29.36874999999999858, 0.000000000000000000, -3.968750000000000000 ) ) ;
#18060=PLANE ( 'NONE',  #6121 ) ;
#18067=CARTESIAN_POINT ( 'NONE',  ( 49.16323787629939801, 32.54502000000000095, -27.09503225884920141 ) ) ;
#18069=EDGE_CURVE ( 'NONE', #19957, #11624, #20033, .T. ) ;
#18075=CARTESIAN_POINT ( 'NONE',  ( 21.43124999999999858, 16.27314499999999953, 10.71562499999999929 ) ) ;
#18086=ORIENTED_EDGE ( 'NONE', *, *, #10629, .T. ) ;
#18097=EDGE_CURVE ( 'NONE', #5953, #17848, #1051, .T. ) ;
#18098=DIRECTION ( 'NONE',  ( 1.000000000000000000, 0.000000000000000000, 0.000000000000000000 ) ) ;
#18109=ORIENTED_EDGE ( 'NONE', *, *, #19537, .F. ) ;
#18115=VERTEX_POINT ( 'NONE', #16531 ) ;
#18120=LINE ( 'NONE', #971, #6503 ) ;
#18121=DIRECTION ( 'NONE',  ( 0.9876802608827760510, 0.000000000000000000, -0.1564854698127960131 ) ) ;
#18124=ORIENTED_EDGE ( 'NONE', *, *, #19528, .T. ) ;
#18126=LINE ( 'NONE', #10934, #19838 ) ;
#18136=ORIENTED_EDGE ( 'NONE', *, *, #2643, .F. ) ;
#18137=DIRECTION ( 'NONE',  ( 0.000000000000000000, 0.000000000000000000, 1.000000000000000000 ) ) ;
#18150=CYLINDRICAL_SURFACE ( 'NONE', #19672, 1.984375000000000000 ) ;
#18151=EDGE_CURVE ( 'NONE', #5739, #11489, #9854, .T. ) ;
#18155=DIRECTION ( 'NONE',  ( -1.000000000000000000, 0.000000000000000000, 0.000000000000000000 ) ) ;
#18163=ORIENTED_EDGE ( 'NONE', *, *, #15908, .F. ) ;
#18165=PRODUCT ( 'Ratchet Main Fixed Frame', 'Ratchet Main Fixed Frame', '', ( #10657 ) ) ;
#18167=DIRECTION ( 'NONE',  ( 1.000000000000000000, 0.000000000000000000, 0.000000000000000000 ) ) ;
#18171=CIRCLE ( 'NONE', #16071, 19.05000000000000071 ) ;
#18193=( NAMED_UNIT ( * ) PLANE_ANGLE_UNIT ( ) SI_UNIT ( $, .RADIAN. ) );
#18194=CIRCLE ( 'NONE', #12180, 0.3962399999999975386 ) ;
#18206=AXIS2_PLACEMENT_3D ( 'NONE', #11909, #16990, #1523 ) ;
#18218=ORIENTED_EDGE ( 'NONE', *, *, #16726, .T. ) ;
#18229=CARTESIAN_POINT ( 'NONE',  ( 2.063750000000000195, 30.56076406250000232, 10.71562496029980061 ) ) ;
#18231=DIRECTION ( 'NONE',  ( 0.000000000000000000, 1.000000000000000000, 0.000000000000000000 ) ) ;
#18234=ORIENTED_EDGE ( 'NONE', *, *, #6183, .T. ) ;
#18238=ORIENTED_EDGE ( 'NONE', *, *, #18993, .F. ) ;
#18248=DIRECTION ( 'NONE',  ( 0.000000000000000000, 1.000000000000000000, 0.000000000000000000 ) ) ;
#18254=DIRECTION ( 'NONE',  ( 0.000000000000000000, 1.000000000000000000, 0.000000000000000000 ) ) ;
#18271=DIRECTION ( 'NONE',  ( 0.000000000000000000, -1.000000000000000000, 0.000000000000000000 ) ) ;
#18272=CARTESIAN_POINT ( 'NONE',  ( -3.929154139288399961, 9.924415000000001541, 0.9374890779182719625 ) ) ;
#18275=VERTEX_POINT ( 'NONE', #11075 ) ;
#18288=CARTESIAN_POINT ( 'NONE',  ( 50.99913033092320092, 0.000000000000000000, -7.029081061492260751 ) ) ;
#18296=ORIENTED_EDGE ( 'NONE', *, *, #5793, .F. ) ;
#18297=CARTESIAN_POINT ( 'NONE',  ( 29.19635173153840313, 30.56064500000000095, -6.218966092919240296 ) ) ;
#18310=DIRECTION ( 'NONE',  ( -0.7776383362760926898, 0.000000000000000000, 0.6287118719681938916 ) ) ;
#18313=ORIENTED_EDGE ( 'NONE', *, *, #10267, .F. ) ;
#18315=ORIENTED_EDGE ( 'NONE', *, *, #16726, .F. ) ;
#18317=CIRCLE ( 'NONE', #12324, 3.968750000000000000 ) ;
#18327=DIRECTION ( 'NONE',  ( 0.000000000000000000, 1.000000000000000000, 0.000000000000000000 ) ) ;
#18328=DIRECTION ( 'NONE',  ( -1.000000000000000000, 0.000000000000000000, 0.000000000000000000 ) ) ;
#18329=DIRECTION ( 'NONE',  ( 1.000000000000000000, 0.000000000000000000, 0.000000000000000000 ) ) ;
#18337=ORIENTED_EDGE ( 'NONE', *, *, #3026, .F. ) ;
#18339=CYLINDRICAL_SURFACE ( 'NONE', #1087, 3.968750000000000000 ) ;
#18348=ORIENTED_EDGE ( 'NONE', *, *, #7224, .F. ) ;
#18351=DIRECTION ( 'NONE',  ( 0.8334497143791951279, 0.000000000000000000, 0.5525953072558960066 ) ) ;
#18354=ORIENTED_EDGE ( 'NONE', *, *, #4095, .T. ) ;
#18363=CARTESIAN_POINT ( 'NONE',  ( 46.03750000000000142, 0.000000000000000000, -10.31874999999999964 ) ) ;
#18377=AXIS2_PLACEMENT_3D ( 'NONE', #6515, #12948, #16475 ) ;
#18390=SHAPE_REPRESENTATION_RELATIONSHIP ( 'NONE' , 'NONE' ,  #21464, #9295 ) ;
#18403=VECTOR ( 'NONE', #9632, 1000.000000000000000 ) ;
#18407=B_SPLINE_CURVE_WITH_KNOTS ( 'NONE', 3,
 ( #7980, #16085, #915, #4459, #17844, #11190, #21351, #4559, #10974, #19478, #21457, #1127, #11299, #7870, #6102, #2789, #18048, #1016, #6316, #5883, #4235, #7763, #12645, #21247, #17728, #2578, #14419, #21134, #5987, #12757, #4349, #14530, #646, #2081, #17463, #7291, #15716, #18992, #873, #12598, #13951, #757, #20649, #20872, #2307, #10822, #9043 ),
 .UNSPECIFIED., .F., .F.,
 ( 4, 1, 1, 1, 1, 1, 1, 1, 1, 1, 1, 1, 1, 1, 1, 1, 1, 1, 1, 1, 1, 1, 1, 1, 1, 1, 1, 1, 1, 1, 1, 1, 1, 1, 1, 1, 1, 1, 1, 1, 1, 1, 1, 1, 4 ),
 ( 0.000000000000000000, 0.02272727272726999745, 0.04545454545455000078, 0.06818181818181999476, 0.09090909090909000956, 0.1136363636363999924, 0.1363636363635999937, 0.1590909090909000123, 0.1818181818182000031, 0.2045454545454999939, 0.2272727272727000092, 0.2500000000000000000, 0.2727272727273000186, 0.2954545454545000061, 0.3181818181818000246, 0.3409090909091000432, 0.3636363636364000063, 0.3863636363635999937, 0.4090909090909000123, 0.4318181818182000309, 0.4545454545454999939, 0.4772727272726999814, 0.5000000000000000000, 0.5227272727273000186, 0.5454545454545000061, 0.5681818181818000246, 0.5909090909091000432, 0.6136363636364000618, 0.6363636363636000493, 0.6590909090908999568, 0.6818181818181999754, 0.7045454545454999939, 0.7272727272726999814, 0.7500000000000000000, 0.7727272727273000186, 0.7954545454545000061, 0.8181818181818000246, 0.8409090909091000432, 0.8636363636364000618, 0.8863636363636000493, 0.9090909090908999568, 0.9318181818181999754, 0.9545454545454999939, 0.9772727272726999814, 1.000000000000000000 ),
 .UNSPECIFIED. ) ;
#18415=ORIENTED_EDGE ( 'NONE', *, *, #6140, .F. ) ;
#18420=DIRECTION ( 'NONE',  ( 0.000000000000000000, 1.000000000000000000, 0.000000000000000000 ) ) ;
#18423=ORIENTED_EDGE ( 'NONE', *, *, #6557, .F. ) ;
#18447=ORIENTED_EDGE ( 'NONE', *, *, #14435, .F. ) ;
#18448=AXIS2_PLACEMENT_3D ( 'NONE', #20845, #20622, #2402 ) ;
#18450=CARTESIAN_POINT ( 'NONE',  ( 21.03437500000000071, 0.000000000000000000, 5.159374999999999822 ) ) ;
#18462=DIRECTION ( 'NONE',  ( 0.000000000000000000, 1.000000000000000000, 0.000000000000000000 ) ) ;
#18468=CARTESIAN_POINT ( 'NONE',  ( 50.99913033092320092, 32.54502000000000095, -7.029081061492260751 ) ) ;
#18476=CARTESIAN_POINT ( 'NONE',  ( 50.99913033092320092, 0.000000000000000000, -7.029081061492260751 ) ) ;
#18479=CARTESIAN_POINT ( 'NONE',  ( -29.36874999999999858, 0.000000000000000000, 10.71562499999999929 ) ) ;
#18481=LINE ( 'NONE', #238, #21866 ) ;
#18489=CARTESIAN_POINT ( 'NONE',  ( 0.02083138522551555155, 12.30439499999999953, 7.210477125664100484 ) ) ;
#18493=CARTESIAN_POINT ( 'NONE',  ( 46.03750000000000142, 0.000000000000000000, -10.31874999999999964 ) ) ;
#18513=DIRECTION ( 'NONE',  ( -1.000000000000000000, 0.000000000000000000, 0.000000000000000000 ) ) ;
#18522=CARTESIAN_POINT ( 'NONE',  ( 23.41562500000000213, 1.984375000000000000, 5.159374999999999822 ) ) ;
#18532=ORIENTED_EDGE ( 'NONE', *, *, #5374, .T. ) ;
#18539=CARTESIAN_POINT ( 'NONE',  ( 26.59062499999999929, 1.984375000000000000, 8.335010000000000474 ) ) ;
#18556=CIRCLE ( 'NONE', #9022, 0.3962399999999998146 ) ;
#18558=CARTESIAN_POINT ( 'NONE',  ( -17.46249999999999858, 16.27314499999999953, 8.731249999999999289 ) ) ;
#18567=ORIENTED_EDGE ( 'NONE', *, *, #4769, .T. ) ;
#18576=VERTEX_POINT ( 'NONE', #13754 ) ;
#18577=ADVANCED_FACE ( 'NONE', ( #18812 ), #12637, .F. ) ;
#18582=DIRECTION ( 'NONE',  ( 0.000000000000000000, 1.000000000000000000, 0.000000000000000000 ) ) ;
#18589=LINE ( 'NONE', #20450, #3700 ) ;
#18590=CARTESIAN_POINT ( 'NONE',  ( 201.9384738932629944, 2.380615000000000148, 8.335010000000000474 ) ) ;
#18604=DIRECTION ( 'NONE',  ( 1.000000000000000000, 0.000000000000000000, 0.000000000000000000 ) ) ;
#18608=CYLINDRICAL_SURFACE ( 'NONE', #16223, 25.00312499999999361 ) ;
#18628=CARTESIAN_POINT ( 'NONE',  ( 54.51779242482700027, 32.54502000000000095, -30.64740209392260084 ) ) ;
#18640=CARTESIAN_POINT ( 'NONE',  ( 1.954387715434429795, 8.736780638212259475, 10.71562499999999929 ) ) ;
#18641=ORIENTED_EDGE ( 'NONE', *, *, #15466, .F. ) ;
#18649=ORIENTED_EDGE ( 'NONE', *, *, #15336, .T. ) ;
#18650=EDGE_CURVE ( 'NONE', #10775, #21819, #10643, .T. ) ;
#18656=ORIENTED_EDGE ( 'NONE', *, *, #14919, .T. ) ;
#18657=CARTESIAN_POINT ( 'NONE',  ( 29.76562500000000000, 0.000000000000000000, -4.317999999999999616 ) ) ;
#18667=VERTEX_POINT ( 'NONE', #19257 ) ;
#18687=FACE_OUTER_BOUND ( 'NONE', #11166, .T. ) ;
#18692=DIRECTION ( 'NONE',  ( 1.000000000000000000, 0.000000000000000000, 0.000000000000000000 ) ) ;
#18698=CARTESIAN_POINT ( 'NONE',  ( 2.063750000000000195, 30.56076406250000232, 10.71562496029980061 ) ) ;
#18709=LINE ( 'NONE', #11980, #13745 ) ;
#18717=AXIS2_PLACEMENT_3D ( 'NONE', #11462, #4604, #14693 ) ;
#18721=EDGE_CURVE ( 'NONE', #16113, #4424, #5658, .T. ) ;
#18724=ADVANCED_FACE ( 'NONE', ( #18920 ), #2236, .F. ) ;
#18727=CARTESIAN_POINT ( 'NONE',  ( 65.90927232300019512, 0.000000000000000000, -13.30734117861468135 ) ) ;
#18735=CARTESIAN_POINT ( 'NONE',  ( 66.03921914090641110, 32.54502000000000095, -11.33033647675950029 ) ) ;
#18741=CIRCLE ( 'NONE', #1082, 9.524999999999998579 ) ;
#18742=AXIS2_PLACEMENT_3D ( 'NONE', #4608, #15020, #11350 ) ;
#18750=PLANE ( 'NONE',  #11750 ) ;
#18756=EDGE_LOOP ( 'NONE', ( #3292, #16220, #20495, #8910 ) ) ;
#18764=AXIS2_PLACEMENT_3D ( 'NONE', #13507, #8188, #18351 ) ;
#18768=VERTEX_POINT ( 'NONE', #11288 ) ;
#18769=CARTESIAN_POINT ( 'NONE',  ( -17.46249999999999858, 0.000000000000000000, 0.000000000000000000 ) ) ;
#18772=VECTOR ( 'NONE', #10830, 1000.000000000000000 ) ;
#18785=DIRECTION ( 'NONE',  ( 0.9579671649362032637, 0.000000000000000000, -0.2868778675745010664 ) ) ;
#18791=ORIENTED_EDGE ( 'NONE', *, *, #12901, .T. ) ;
#18793=ORIENTED_EDGE ( 'NONE', *, *, #3188, .F. ) ;
#18796=CIRCLE ( 'NONE', #19152, 1.984374999999998890 ) ;
#18801=CARTESIAN_POINT ( 'NONE',  ( 67.40134256979101224, 1.984375000000000000, -13.70358117861468017 ) ) ;
#18809=VECTOR ( 'NONE', #16420, 1000.000000000000000 ) ;
#18812=FACE_OUTER_BOUND ( 'NONE', #1164, .T. ) ;
#18819=CIRCLE ( 'NONE', #4020, 0.3962399999999999811 ) ;
#18852=ORIENTED_EDGE ( 'NONE', *, *, #21666, .T. ) ;
#18856=ADVANCED_FACE ( 'NONE', ( #2894 ), #2780, .F. ) ;
#18857=DIRECTION ( 'NONE',  ( 0.000000000000000000, -1.000000000000000000, 0.000000000000000000 ) ) ;
#18861=VERTEX_POINT ( 'NONE', #19900 ) ;
#18862=AXIS2_PLACEMENT_3D ( 'NONE', #1668, #11959, #11856 ) ;
#18873=CARTESIAN_POINT ( 'NONE',  ( -20.63749999999999929, 16.27314499999999953, 8.731249999999999289 ) ) ;
#18876=ORIENTED_EDGE ( 'NONE', *, *, #13563, .T. ) ;
#18886=AXIS2_PLACEMENT_3D ( 'NONE', #16206, #2702, #15573 ) ;
#18887=ORIENTED_EDGE ( 'NONE', *, *, #6650, .T. ) ;
#18889=CARTESIAN_POINT ( 'NONE',  ( 67.40134256979101224, 74.97070807199999365, -13.70358117861468017 ) ) ;
#18899=ORIENTED_EDGE ( 'NONE', *, *, #7242, .T. ) ;
#18905=EDGE_CURVE ( 'NONE', #17225, #10798, #15253, .T. ) ;
#18913=EDGE_CURVE ( 'NONE', #13013, #3881, #15262, .T. ) ;
#18920=FACE_OUTER_BOUND ( 'NONE', #15457, .T. ) ;
#18936=ORIENTED_EDGE ( 'NONE', *, *, #4097, .T. ) ;
#18940=LINE ( 'NONE', #14224, #436 ) ;
#18944=UNCERTAINTY_MEASURE_WITH_UNIT (LENGTH_MEASURE( 1.000000000000000082E-05 ), #20231, 'distance_accuracy_value', 'NONE');
#18954=ADVANCED_FACE ( 'NONE', ( #20319 ), #1553, .T. ) ;
#18957=EDGE_LOOP ( 'NONE', ( #21562, #1179, #8675, #4233 ) ) ;
#18959=CYLINDRICAL_SURFACE ( 'NONE', #7707, 0.7950200000000005041 ) ;
#18972=VERTEX_POINT ( 'NONE', #9953 ) ;
#18975=DIRECTION ( 'NONE',  ( 1.000000000000000000, 0.000000000000000000, 0.000000000000000000 ) ) ;
#18987=ORIENTED_EDGE ( 'NONE', *, *, #7734, .T. ) ;
#18990=VERTEX_POINT ( 'NONE', #15166 ) ;
#18992=CARTESIAN_POINT ( 'NONE',  ( 13.01576158600160049, 0.2519556637135220156, 9.701108553893439179 ) ) ;
#18993=EDGE_CURVE ( 'NONE', #20988, #4180, #20156, .T. ) ;
#18995=CARTESIAN_POINT ( 'NONE',  ( 49.81956284419040060, 1.984375000000000000, 11.98436472153758103 ) ) ;
#18998=CARTESIAN_POINT ( 'NONE',  ( 0.000000000000000000, 32.54502000000000095, 0.000000000000000000 ) ) ;
#19004=ORIENTED_EDGE ( 'NONE', *, *, #2770, .F. ) ;
#19017=DIRECTION ( 'NONE',  ( 0.000000000000000000, 0.000000000000000000, 1.000000000000000000 ) ) ;
#19038=DIRECTION ( 'NONE',  ( 0.000000000000000000, 1.000000000000000000, 0.000000000000000000 ) ) ;
#19042=FACE_BOUND ( 'NONE', #8275, .T. ) ;
#19050=EDGE_CURVE ( 'NONE', #11624, #14525, #46, .T. ) ;
#19053=FACE_OUTER_BOUND ( 'NONE', #15618, .T. ) ;
#19077=ADVANCED_FACE ( 'NONE', ( #16603 ), #15067, .T. ) ;
#19080=DIRECTION ( 'NONE',  ( 0.000000000000000000, 1.000000000000000000, 0.000000000000000000 ) ) ;
#19095=CIRCLE ( 'NONE', #4631, 2.381250000000001421 ) ;
#19099=ORIENTED_EDGE ( 'NONE', *, *, #7404, .F. ) ;
#19105=VECTOR ( 'NONE', #21738, 1000.000000000000000 ) ;
#19124=VERTEX_POINT ( 'NONE', #21782 ) ;
#19126=VERTEX_POINT ( 'NONE', #16812 ) ;
#19127=CARTESIAN_POINT ( 'NONE',  ( 46.03750000000000142, 32.54502000000000095, -10.31874999999999964 ) ) ;
#19128=VECTOR ( 'NONE', #8725, 1000.000000000000000 ) ;
#19142=AXIS2_PLACEMENT_3D ( 'NONE', #1252, #15089, #21590 ) ;
#19152=AXIS2_PLACEMENT_3D ( 'NONE', #10906, #17655, #5919 ) ;
#19160=ORIENTED_EDGE ( 'NONE', *, *, #17583, .F. ) ;
#19167=ORIENTED_EDGE ( 'NONE', *, *, #10744, .T. ) ;
#19168=VECTOR ( 'NONE', #15306, 1000.000000000000227 ) ;
#19181=DIRECTION ( 'NONE',  ( 0.000000000000000000, 1.000000000000000000, 0.000000000000000000 ) ) ;
#19183=FACE_OUTER_BOUND ( 'NONE', #11215, .T. ) ;
#19203=LINE ( 'NONE', #630, #4509 ) ;
#19205=ORIENTED_EDGE ( 'NONE', *, *, #4095, .F. ) ;
#19212=ORIENTED_EDGE ( 'NONE', *, *, #20237, .F. ) ;
#19219=CARTESIAN_POINT ( 'NONE',  ( -29.36874999999999858, 30.56064500000000095, -3.968750000000000000 ) ) ;
#19221=CARTESIAN_POINT ( 'NONE',  ( 1.405219880766735541, 23.42673279364623085, 8.655316695198486343 ) ) ;
#19222=CARTESIAN_POINT ( 'NONE',  ( 49.41235866845560309, 0.000000000000000000, -26.78690084448080100 ) ) ;
#19229=CARTESIAN_POINT ( 'NONE',  ( 6.585898268469219552, 1.984375000000000000, 4.694966092919240275 ) ) ;
#19230=PLANE ( 'NONE',  #67 ) ;
#19239=AXIS2_PLACEMENT_3D ( 'NONE', #1084, #8154, #18121 ) ;
#19240=ORIENTED_EDGE ( 'NONE', *, *, #7760, .T. ) ;
#19244=LINE ( 'NONE', #15740, #3117 ) ;
#19245=EDGE_CURVE ( 'NONE', #12825, #9456, #2165, .T. ) ;
#19254=CARTESIAN_POINT ( 'NONE',  ( 70.64340948846358970, 0.000000000000000000, -10.93409647675949969 ) ) ;
#19257=CARTESIAN_POINT ( 'NONE',  ( 23.41562500000000213, 32.54502000000000095, 5.159374999999999822 ) ) ;
#19258=CARTESIAN_POINT ( 'NONE',  ( 26.59062499999999929, 30.16440499999999858, 8.731249999999999289 ) ) ;
#19271=CARTESIAN_POINT ( 'NONE',  ( 0.05261182704408059324, 23.41816500000000190, 7.316601101023040066 ) ) ;
#19275=VERTEX_POINT ( 'NONE', #2089 ) ;
#19297=EDGE_LOOP ( 'NONE', ( #13253, #1550, #14021, #21305 ) ) ;
#19301=ORIENTED_EDGE ( 'NONE', *, *, #14384, .T. ) ;
#19308=CARTESIAN_POINT ( 'NONE',  ( 71.04062499999999147, 30.56064500000000095, -10.31874999999999964 ) ) ;
#19310=CARTESIAN_POINT ( 'NONE',  ( 54.51779242482700027, 32.54502000000000095, -30.64740209392260084 ) ) ;
#19321=ORIENTED_EDGE ( 'NONE', *, *, #3026, .T. ) ;
#19323=DIRECTION ( 'NONE',  ( -0.5733392046337749681, 0.8193181045417647912, 0.000000000000000000 ) ) ;
#19326=EDGE_CURVE ( 'NONE', #17848, #13038, #16258, .T. ) ;
#19327=VECTOR ( 'NONE', #14846, 1000.000000000000000 ) ;
#19328=VERTEX_POINT ( 'NONE', #1204 ) ;
#19333=VERTEX_POINT ( 'NONE', #7947 ) ;
#19337=LINE ( 'NONE', #2761, #411 ) ;
#19339=ORIENTED_EDGE ( 'NONE', *, *, #21306, .T. ) ;
#19359=LINE ( 'NONE', #15752, #8222 ) ;
#19362=LINE ( 'NONE', #2570, #10662 ) ;
#19369=CARTESIAN_POINT ( 'NONE',  ( 54.11611804786240043, 0.000000000000000000, -30.58983753981140197 ) ) ;
#19389=ORIENTED_EDGE ( 'NONE', *, *, #2643, .T. ) ;
#19390=ORIENTED_EDGE ( 'NONE', *, *, #12516, .T. ) ;
#19394=CARTESIAN_POINT ( 'NONE',  ( -12.30312499606204035, 30.56080375000000160, 10.71562494918373964 ) ) ;
#19396=DIRECTION ( 'NONE',  ( 0.000000000000000000, 1.000000000000000000, 0.000000000000000000 ) ) ;
#19400=CARTESIAN_POINT ( 'NONE',  ( 5.447351731530780228, 32.54502000000000095, 0.8930339070797439494 ) ) ;
#19409=ORIENTED_EDGE ( 'NONE', *, *, #2108, .T. ) ;
#19414=LINE ( 'NONE', #5829, #8376 ) ;
#19415=ORIENTED_EDGE ( 'NONE', *, *, #16529, .T. ) ;
#19425=EDGE_CURVE ( 'NONE', #15199, #1402, #18126, .T. ) ;
#19428=AXIS2_PLACEMENT_3D ( 'NONE', #7675, #12779, #19502 ) ;
#19431=AXIS2_PLACEMENT_3D ( 'NONE', #4949, #10370, #11817 ) ;
#19439=CYLINDRICAL_SURFACE ( 'NONE', #1139, 3.175000000000000711 ) ;
#19440=CARTESIAN_POINT ( 'NONE',  ( -17.46249999999999858, 30.56064500000000095, 0.000000000000000000 ) ) ;
#19441=ORIENTED_EDGE ( 'NONE', *, *, #14796, .T. ) ;
#19458=CIRCLE ( 'NONE', #17299, 16.66874999999998508 ) ;
#19473=CYLINDRICAL_SURFACE ( 'NONE', #5315, 0.7950200000000005041 ) ;
#19474=VECTOR ( 'NONE', #10859, 1000.000000000000000 ) ;
#19478=CARTESIAN_POINT ( 'NONE',  ( 28.63992156299379843, 1.561888874053700027, 10.67040950666179988 ) ) ;
#19489=FACE_OUTER_BOUND ( 'NONE', #3163, .T. ) ;
#19493=ORIENTED_EDGE ( 'NONE', *, *, #6160, .T. ) ;
#19502=DIRECTION ( 'NONE',  ( 1.000000000000000000, 0.000000000000000000, 0.000000000000000000 ) ) ;
#19510=DIRECTION ( 'NONE',  ( 0.000000000000000000, -1.000000000000000000, 0.000000000000000000 ) ) ;
#19519=CARTESIAN_POINT ( 'NONE',  ( 1.719806708599410427, 8.992310301660250360, 8.718447211008458098 ) ) ;
#19522=EDGE_CURVE ( 'NONE', #7142, #4736, #2905, .T. ) ;
#19525=EDGE_LOOP ( 'NONE', ( #1838, #11258, #17204, #14682 ) ) ;
#19528=EDGE_CURVE ( 'NONE', #11564, #20988, #14571, .T. ) ;
#19537=EDGE_CURVE ( 'NONE', #8141, #9016, #3249, .T. ) ;
#19545=VERTEX_POINT ( 'NONE', #10141 ) ;
#19546=ORIENTED_EDGE ( 'NONE', *, *, #15072, .F. ) ;
#19547=AXIS2_PLACEMENT_3D ( 'NONE', #18801, #20902, #19017 ) ;
#19555=ORIENTED_EDGE ( 'NONE', *, *, #20284, .F. ) ;
#19559=CYLINDRICAL_SURFACE ( 'NONE', #10559, 3.175000000000000711 ) ;
#19564=CARTESIAN_POINT ( 'NONE',  ( 46.03750000000000142, 30.56064500000000095, -10.31874999999999964 ) ) ;
#19585=DIRECTION ( 'NONE',  ( 0.000000000000000000, -1.000000000000000000, 0.000000000000000000 ) ) ;
#19589=ADVANCED_FACE ( 'NONE', ( #16790 ), #6833, .T. ) ;
#19591=VERTEX_POINT ( 'NONE', #3513 ) ;
#19595=CARTESIAN_POINT ( 'NONE',  ( -17.46249999999999858, 32.54502000000000095, 0.000000000000000000 ) ) ;
#19597=EDGE_LOOP ( 'NONE', ( #7399, #10679, #12364, #12701, #20745, #5169 ) ) ;
#19616=DIRECTION ( 'NONE',  ( -0.6287118719681975554, 0.000000000000000000, -0.7776383362760898033 ) ) ;
#19625=CARTESIAN_POINT ( 'NONE',  ( 49.41235866845560309, 30.56064500000000095, -26.78690084448080100 ) ) ;
#19632=DIRECTION ( 'NONE',  ( 1.000000000000000000, 0.000000000000000000, 0.000000000000000000 ) ) ;
#19633=ORIENTED_EDGE ( 'NONE', *, *, #14413, .F. ) ;
#19634=EDGE_LOOP ( 'NONE', ( #14622, #21297, #13278, #11924 ) ) ;
#19638=ORIENTED_EDGE ( 'NONE', *, *, #4798, .F. ) ;
#19648=LINE ( 'NONE', #21312, #2998 ) ;
#19656=DIRECTION ( 'NONE',  ( 0.000000000000000000, 0.000000000000000000, -1.000000000000000000 ) ) ;
#19672=AXIS2_PLACEMENT_3D ( 'NONE', #19896, #14959, #14739 ) ;
#19674=CARTESIAN_POINT ( 'NONE',  ( 28.97711086133420366, 0.000000000000000000, -10.71499000000000024 ) ) ;
#19683=VERTEX_POINT ( 'NONE', #13275 ) ;
#19695=CARTESIAN_POINT ( 'NONE',  ( 54.29867169743560140, 0.000000000000000000, -30.73743011777780154 ) ) ;
#19711=ORIENTED_EDGE ( 'NONE', *, *, #6557, .T. ) ;
#19713=CARTESIAN_POINT ( 'NONE',  ( 46.03750000000000142, 1.984375000000000000, -10.31874999999999964 ) ) ;
#19714=LINE ( 'NONE', #13429, #15649 ) ;
#19716=DIRECTION ( 'NONE',  ( 0.000000000000000000, -1.000000000000000000, 0.000000000000000000 ) ) ;
#19718=CYLINDRICAL_SURFACE ( 'NONE', #10988, 1.984375000000000888 ) ;
#19727=VECTOR ( 'NONE', #12147, 1000.000000000000000 ) ;
#19728=CARTESIAN_POINT ( 'NONE',  ( 46.03750000000000142, 1.984375000000000000, -10.31874999999999964 ) ) ;
#19735=ORIENTED_EDGE ( 'NONE', *, *, #4239, .T. ) ;
#19739=DIRECTION ( 'NONE',  ( 0.000000000000000000, -1.000000000000000000, 0.000000000000000000 ) ) ;
#19746=VERTEX_POINT ( 'NONE', #20515 ) ;
#19784=FACE_OUTER_BOUND ( 'NONE', #21789, .T. ) ;
#19791=CARTESIAN_POINT ( 'NONE',  ( -12.30312499999999964, 1.984375000000000000, 8.731249999999999289 ) ) ;
#19799=CIRCLE ( 'NONE', #10269, 0.3962399999999998146 ) ;
#19801=DIRECTION ( 'NONE',  ( -1.000000000000000000, 0.000000000000000000, 0.000000000000000000 ) ) ;
#19804=SURFACE_SIDE_STYLE ('',( #21463 ) ) ;
#19810=VECTOR ( 'NONE', #9262, 1000.000000000000000 ) ;
#19811=LINE ( 'NONE', #6445, #3171 ) ;
#19815=VECTOR ( 'NONE', #7408, 1000.000000000000227 ) ;
#19816=CARTESIAN_POINT ( 'NONE',  ( 49.09065990372640442, 1.984375000000000000, -26.70549589918839928 ) ) ;
#19828=CARTESIAN_POINT ( 'NONE',  ( 65.90927232300019512, 30.56064500000000095, -12.91110117861467899 ) ) ;
#19831=CARTESIAN_POINT ( 'NONE',  ( 28.97711086133420366, 1.984375000000000000, -10.71499000000000024 ) ) ;
#19834=DIRECTION ( 'NONE',  ( 0.000000000000000000, 1.000000000000000000, 0.000000000000000000 ) ) ;
#19838=VECTOR ( 'NONE', #5948, 1000.000000000000000 ) ;
#19845=VECTOR ( 'NONE', #16680, 1000.000000000000000 ) ;
#19847=CYLINDRICAL_SURFACE ( 'NONE', #15931, 3.968750000000000000 ) ;
#19851=ORIENTED_EDGE ( 'NONE', *, *, #5878, .T. ) ;
#19854=VECTOR ( 'NONE', #19181, 1000.000000000000000 ) ;
#19856=AXIS2_PLACEMENT_3D ( 'NONE', #17524, #10547, #4251 ) ;
#19863=AXIS2_PLACEMENT_3D ( 'NONE', #7946, #16257, #16364 ) ;
#19865=VERTEX_POINT ( 'NONE', #2178 ) ;
#19872=ORIENTED_EDGE ( 'NONE', *, *, #19905, .T. ) ;
#19874=DIRECTION ( 'NONE',  ( 0.000000000000000000, 1.000000000000000000, 0.000000000000000000 ) ) ;
#19878=ORIENTED_EDGE ( 'NONE', *, *, #10197, .F. ) ;
#19885=ORIENTED_EDGE ( 'NONE', *, *, #1086, .F. ) ;
#19887=CARTESIAN_POINT ( 'NONE',  ( -21.43124999999999858, 0.000000000000000000, -4.860316984116058095E-16 ) ) ;
#19896=CARTESIAN_POINT ( 'NONE',  ( 29.76562500000000000, 32.54502000000000095, -4.317999999999999616 ) ) ;
#19897=ORIENTED_EDGE ( 'NONE', *, *, #10953, .T. ) ;
#19899=CIRCLE ( 'NONE', #1552, 2.381250000000001421 ) ;
#19900=CARTESIAN_POINT ( 'NONE',  ( 65.64431122251959039, 30.56064500000000095, -11.29787305743958115 ) ) ;
#19905=EDGE_CURVE ( 'NONE', #17319, #15944, #3961, .T. ) ;
#19914=CARTESIAN_POINT ( 'NONE',  ( 201.9384738932629944, 2.380615000000000148, 8.335010000000000474 ) ) ;
#19922=DIRECTION ( 'NONE',  ( 0.000000000000000000, 0.000000000000000000, 1.000000000000000000 ) ) ;
#19943=CARTESIAN_POINT ( 'NONE',  ( 29.37324403177899868, 0.000000000000000000, -10.70578951775076071 ) ) ;
#19957=VERTEX_POINT ( 'NONE', #16426 ) ;
#19965=CARTESIAN_POINT ( 'NONE',  ( 2.063750000000000195, 8.334374999999999645, 10.71562499999999929 ) ) ;
#19966=ORIENTED_EDGE ( 'NONE', *, *, #5898, .T. ) ;
#19975=CARTESIAN_POINT ( 'NONE',  ( -12.30312499999999964, 30.56064500000000095, 8.335010000000000474 ) ) ;
#19987=CARTESIAN_POINT ( 'NONE',  ( 23.41562500000000213, 32.54502000000000095, 5.159374999999999822 ) ) ;
#19995=CARTESIAN_POINT ( 'NONE',  ( 46.03750000000000142, 30.56064500000000095, -10.31874999999999964 ) ) ;
#20000=ORIENTED_EDGE ( 'NONE', *, *, #2108, .F. ) ;
#20003=CARTESIAN_POINT ( 'NONE',  ( -13.49374999999999858, 0.000000000000000000, 0.000000000000000000 ) ) ;
#20015=FACE_OUTER_BOUND ( 'NONE', #6608, .T. ) ;
#20025=DIRECTION ( 'NONE',  ( 0.000000000000000000, -1.000000000000000000, 0.000000000000000000 ) ) ;
#20030=CARTESIAN_POINT ( 'NONE',  ( -2.607150795738780058, 0.000000000000000000, 8.731885000000000119 ) ) ;
#20033=LINE ( 'NONE', #11444, #16934 ) ;
#20035=LINE ( 'NONE', #6238, #3175 ) ;
#20045=VERTEX_POINT ( 'NONE', #20030 ) ;
#20062=DIRECTION ( 'NONE',  ( -0.9579671649362033747, 0.000000000000000000, 0.2868778675745011220 ) ) ;
#20072=DIRECTION ( 'NONE',  ( 0.9579671649362032637, 0.000000000000000000, -0.2868778675745010664 ) ) ;
#20076=DIRECTION ( 'NONE',  ( 0.1831666983862991482, 0.000000000000000000, -0.9830818687180954418 ) ) ;
#20077=CARTESIAN_POINT ( 'NONE',  ( 29.36874999999999858, 9.921875000000000000, 8.731249999999999289 ) ) ;
#20083=CARTESIAN_POINT ( 'NONE',  ( 26.59062499999999929, 1.984375000000000000, 8.335010000000000474 ) ) ;
#20094=CARTESIAN_POINT ( 'NONE',  ( 29.76562500000000000, 30.56064500000000095, -4.317999999999999616 ) ) ;
#20111=ORIENTED_EDGE ( 'NONE', *, *, #16264, .F. ) ;
#20117=AXIS2_PLACEMENT_3D ( 'NONE', #3554, #10293, #21793 ) ;
#20121=AXIS2_PLACEMENT_3D ( 'NONE', #18735, #507, #15677 ) ;
#20131=VECTOR ( 'NONE', #21546, 1000.000000000000114 ) ;
#20143=DIRECTION ( 'NONE',  ( 0.000000000000000000, 0.000000000000000000, -1.000000000000000000 ) ) ;
#20154=CARTESIAN_POINT ( 'NONE',  ( -1.880134707694870011, 12.30439499999999953, 7.779750394130780400 ) ) ;
#20156=CIRCLE ( 'NONE', #18764, 25.00312500000000426 ) ;
#20157=ADVANCED_FACE ( 'NONE', ( #4704 ), #9994, .T. ) ;
#20164=VERTEX_POINT ( 'NONE', #1686 ) ;
#20165=ORIENTED_EDGE ( 'NONE', *, *, #5199, .T. ) ;
#20172=FACE_OUTER_BOUND ( 'NONE', #16088, .T. ) ;
#20173=EDGE_LOOP ( 'NONE', ( #13551, #6576, #11238, #14316 ) ) ;
#20178=VECTOR ( 'NONE', #7200, 1000.000000000000000 ) ;
#20185=LINE ( 'NONE', #18539, #1156 ) ;
#20190=EDGE_CURVE ( 'NONE', #3431, #14260, #1145, .T. ) ;
#20196=FACE_BOUND ( 'NONE', #12255, .T. ) ;
#20206=ORIENTED_EDGE ( 'NONE', *, *, #8308, .F. ) ;
#20207=DIRECTION ( 'NONE',  ( 0.000000000000000000, 0.000000000000000000, -1.000000000000000000 ) ) ;
#20212=CARTESIAN_POINT ( 'NONE',  ( 6.585898268469219552, 32.54502000000000095, 4.694966092919240275 ) ) ;
#20213=FACE_OUTER_BOUND ( 'NONE', #13688, .T. ) ;
#20216=CARTESIAN_POINT ( 'NONE',  ( 2.063750000000000195, 30.56064500000000095, -5.492750000000000021 ) ) ;
#20219=CARTESIAN_POINT ( 'NONE',  ( 6.016625000000000334, 0.000000000000000000, 2.794000000000000039 ) ) ;
#20231=( LENGTH_UNIT ( ) NAMED_UNIT ( * ) SI_UNIT ( .MILLI., .METRE. ) );
#20233=DIRECTION ( 'NONE',  ( 0.000000000000000000, 0.000000000000000000, -1.000000000000000000 ) ) ;
#20237=EDGE_CURVE ( 'NONE', #4424, #2932, #19714, .T. ) ;
#20255=CARTESIAN_POINT ( 'NONE',  ( 2.063749999357820109, 1.984315468747399835, 10.71562492933363941 ) ) ;
#20270=AXIS2_PLACEMENT_3D ( 'NONE', #13721, #5284, #7066 ) ;
#20282=LINE ( 'NONE', #3835, #14180 ) ;
#20283=ORIENTED_EDGE ( 'NONE', *, *, #20237, .T. ) ;
#20284=EDGE_CURVE ( 'NONE', #3881, #4736, #20492, .T. ) ;
#20285=ADVANCED_FACE ( 'NONE', ( #6915 ), #20829, .F. ) ;
#20286=EDGE_CURVE ( 'NONE', #19683, #14134, #20722, .T. ) ;
#20292=ORIENTED_EDGE ( 'NONE', *, *, #8979, .F. ) ;
#20296=DIRECTION ( 'NONE',  ( -1.000000000000000000, 0.000000000000000000, 0.000000000000000000 ) ) ;
#20299=ORIENTED_EDGE ( 'NONE', *, *, #14538, .F. ) ;
#20312=DIRECTION ( 'NONE',  ( 0.000000000000000000, 1.000000000000000000, 0.000000000000000000 ) ) ;
#20316=LINE ( 'NONE', #10164, #9086 ) ;
#20319=FACE_OUTER_BOUND ( 'NONE', #5254, .T. ) ;
#20336=CARTESIAN_POINT ( 'NONE',  ( 16.12871017875626478, 32.54500158971978863, 9.894232675333643812 ) ) ;
#20355=DIRECTION ( 'NONE',  ( -0.06191955310929838502, 0.000000000000000000, 0.9980811434661737147 ) ) ;
#20358=CARTESIAN_POINT ( 'NONE',  ( 2.063750000000000195, 8.334374999999999645, 8.731249999999999289 ) ) ;
#20363=ORIENTED_EDGE ( 'NONE', *, *, #6431, .F. ) ;
#20389=PRODUCT_DEFINITION_FORMATION_WITH_SPECIFIED_SOURCE ( 'ANY', '', #18165, .NOT_KNOWN. ) ;
#20393=PLANE ( 'NONE',  #6190 ) ;
#20400=FACE_OUTER_BOUND ( 'NONE', #16686, .T. ) ;
#20407=ORIENTED_EDGE ( 'NONE', *, *, #6206, .F. ) ;
#20408=ORIENTED_EDGE ( 'NONE', *, *, #5034, .T. ) ;
#20409=DIRECTION ( 'NONE',  ( 0.000000000000000000, 1.000000000000000000, 0.000000000000000000 ) ) ;
#20414=AXIS2_PLACEMENT_3D ( 'NONE', #17557, #15804, #7378 ) ;
#20420=ORIENTED_EDGE ( 'NONE', *, *, #6904, .F. ) ;
#20425=EDGE_CURVE ( 'NONE', #2020, #138, #717, .T. ) ;
#20429=CYLINDRICAL_SURFACE ( 'NONE', #20512, 1.984375000000000000 ) ;
#20442=AXIS2_PLACEMENT_3D ( 'NONE', #10205, #20355, #11982 ) ;
#20450=CARTESIAN_POINT ( 'NONE',  ( 29.36874999999999858, 9.921875000000000000, 10.71562499999999929 ) ) ;
#20471=AXIS2_PLACEMENT_3D ( 'NONE', #14201, #12198, #17604 ) ;
#20480=CIRCLE ( 'NONE', #10978, 0.3962400000000008138 ) ;
#20486=ORIENTED_EDGE ( 'NONE', *, *, #21280, .T. ) ;
#20492=LINE ( 'NONE', #3937, #19854 ) ;
#20495=ORIENTED_EDGE ( 'NONE', *, *, #6294, .F. ) ;
#20499=CIRCLE ( 'NONE', #4986, 16.66874999999998508 ) ;
#20507=CARTESIAN_POINT ( 'NONE',  ( 6.585898268469219552, 32.54502000000000095, 4.694966092919240275 ) ) ;
#20510=CARTESIAN_POINT ( 'NONE',  ( 1.336161662408851036, 9.129395000000000593, 10.66779089274961123 ) ) ;
#20512=AXIS2_PLACEMENT_3D ( 'NONE', #7205, #3883, #17370 ) ;
#20515=CARTESIAN_POINT ( 'NONE',  ( 18.65312499999999929, 1.984375000000000000, 5.159374999999999822 ) ) ;
#20517=DIRECTION ( 'NONE',  ( 0.8334497143791951279, 0.000000000000000000, 0.5525953072558960066 ) ) ;
#20520=ORIENTED_EDGE ( 'NONE', *, *, #2336, .F. ) ;
#20528=DIRECTION ( 'NONE',  ( 0.2868778675745004558, 0.000000000000000000, 0.9579671649362035968 ) ) ;
#20531=VECTOR ( 'NONE', #17105, 1000.000000000000000 ) ;
#20538=CARTESIAN_POINT ( 'NONE',  ( 49.16323787629939801, -42.42568807200000691, -27.09503225884920141 ) ) ;
#20540=EDGE_CURVE ( 'NONE', #18861, #3318, #1972, .T. ) ;
#20547=CIRCLE ( 'NONE', #10695, 1.984374999999998890 ) ;
#20550=CARTESIAN_POINT ( 'NONE',  ( -12.30312499999999964, 30.16440499999999858, 8.731249999999999289 ) ) ;
#20557=AXIS2_PLACEMENT_3D ( 'NONE', #12682, #2504, #15907 ) ;
#20559=LINE ( 'NONE', #7533, #10158 ) ;
#20563=VECTOR ( 'NONE', #14518, 1000.000000000000000 ) ;
#20573=DIRECTION ( 'NONE',  ( 0.9999999999672709583, 8.090614674031770259E-06, 1.618640956562950034E-09 ) ) ;
#20577=CARTESIAN_POINT ( 'NONE',  ( 21.43124999999999858, 16.27314499999999953, 8.731249999999999289 ) ) ;
#20590=CARTESIAN_POINT ( 'NONE',  ( 6.585898268469219552, 0.000000000000000000, 4.694966092919240275 ) ) ;
#20596=VECTOR ( 'NONE', #214, 1000.000000000000000 ) ;
#20602=LINE ( 'NONE', #2146, #3548 ) ;
#20606=VECTOR ( 'NONE', #11610, 1000.000000000000000 ) ;
#20612=FACE_OUTER_BOUND ( 'NONE', #7117, .T. ) ;
#20613=VERTEX_POINT ( 'NONE', #1469 ) ;
#20618=CARTESIAN_POINT ( 'NONE',  ( 49.81956284419040060, 0.000000000000000000, 11.98436472153758103 ) ) ;
#20619=ORIENTED_EDGE ( 'NONE', *, *, #7760, .F. ) ;
#20622=DIRECTION ( 'NONE',  ( 0.000000000000000000, 1.000000000000000000, 0.000000000000000000 ) ) ;
#20625=CARTESIAN_POINT ( 'NONE',  ( 29.19635173153840313, 1.984375000000000000, -6.218966092919240296 ) ) ;
#20630=DIRECTION ( 'NONE',  ( -1.000000000000000000, 0.000000000000000000, 0.000000000000000000 ) ) ;
#20637=CARTESIAN_POINT ( 'NONE',  ( -23.01875000000000071, 1.984375000000000000, -10.31874999999999964 ) ) ;
#20649=CARTESIAN_POINT ( 'NONE',  ( 4.479823106602060179, 0.04783660261014419796, 9.171550912739061090 ) ) ;
#20685=DIRECTION ( 'NONE',  ( 0.000000000000000000, 0.000000000000000000, 1.000000000000000000 ) ) ;
#20686=FACE_OUTER_BOUND ( 'NONE', #1503, .T. ) ;
#20702=EDGE_CURVE ( 'NONE', #3268, #11564, #15631, .T. ) ;
#20703=LINE ( 'NONE', #20590, #10049 ) ;
#20717=EDGE_CURVE ( 'NONE', #15983, #20613, #8395, .T. ) ;
#20719=ORIENTED_EDGE ( 'NONE', *, *, #16678, .T. ) ;
#20722=LINE ( 'NONE', #8569, #3623 ) ;
#20733=ORIENTED_EDGE ( 'NONE', *, *, #4842, .T. ) ;
#20740=CARTESIAN_POINT ( 'NONE',  ( 54.11611804786240043, 32.54502000000000095, -30.58983753981140197 ) ) ;
#20745=ORIENTED_EDGE ( 'NONE', *, *, #1543, .T. ) ;
#20750=AXIS2_PLACEMENT_3D ( 'NONE', #18363, #1771, #7087 ) ;
#20768=DIRECTION ( 'NONE',  ( -1.000000000000000000, 0.000000000000000000, 0.000000000000000000 ) ) ;
#20770=FACE_BOUND ( 'NONE', #9335, .T. ) ;
#20771=ORIENTED_EDGE ( 'NONE', *, *, #7225, .F. ) ;
#20787=DIRECTION ( 'NONE',  ( 0.000000000000000000, 1.000000000000000000, 0.000000000000000000 ) ) ;
#20791=CARTESIAN_POINT ( 'NONE',  ( 26.59062499999999929, 1.984375000000000000, 8.731249999999999289 ) ) ;
#20796=LINE ( 'NONE', #17399, #9218 ) ;
#20804=DIRECTION ( 'NONE',  ( 0.000000000000000000, -1.000000000000000000, 0.000000000000000000 ) ) ;
#20811=ORIENTED_EDGE ( 'NONE', *, *, #7352, .T. ) ;
#20821=COLOUR_RGB ( '', 0.72549020, 0.75294118, 0.79215686) ;
#20829=CYLINDRICAL_SURFACE ( 'NONE', #11742, 1.984375000000000000 ) ;
#20835=CARTESIAN_POINT ( 'NONE',  ( 1.406764971174492729, 9.129395000000000593, 8.660233583965718296 ) ) ;
#20837=CARTESIAN_POINT ( 'NONE',  ( 29.19635173153840313, 32.54502000000000095, -6.218966092919240296 ) ) ;
#20845=CARTESIAN_POINT ( 'NONE',  ( 46.03750000000000142, 0.000000000000000000, -10.31874999999999964 ) ) ;
#20846=LINE ( 'NONE', #1061, #10500 ) ;
#20853=DIRECTION ( 'NONE',  ( 0.000000000000000000, -1.000000000000000000, 0.000000000000000000 ) ) ;
#20856=ORIENTED_EDGE ( 'NONE', *, *, #2974, .F. ) ;
#20860=VECTOR ( 'NONE', #19739, 1000.000000000000000 ) ;
#20867=EDGE_CURVE ( 'NONE', #18768, #4510, #2091, .T. ) ;
#20872=CARTESIAN_POINT ( 'NONE',  ( 2.318742500528585104, 0.02198808074787805128, 9.037480505500679939 ) ) ;
#20881=CARTESIAN_POINT ( 'NONE',  ( 65.90927232300019512, 0.000000000000000000, -13.30734117861468135 ) ) ;
#20885=( BOUNDED_CURVE ( )  B_SPLINE_CURVE ( 3, ( #8313, #20336, #11961, #12626 ),
 .UNSPECIFIED., .F., .T. ) 
 B_SPLINE_CURVE_WITH_KNOTS ( ( 4, 4 ),
 ( 4.712488883238074244, 6.283478609653115221 ),
 .UNSPECIFIED. ) 
 CURVE ( )  GEOMETRIC_REPRESENTATION_ITEM ( )  RATIONAL_B_SPLINE_CURVE ( ( 1.000000000000000000, 0.8046922671927911885, 0.8046922671927911885, 1.000000000000000000 ) ) 
 REPRESENTATION_ITEM ( '' )  );
#20889=ORIENTED_EDGE ( 'NONE', *, *, #21663, .T. ) ;
#20891=VERTEX_POINT ( 'NONE', #20881 ) ;
#20900=VECTOR ( 'NONE', #18785, 1000.000000000000227 ) ;
#20902=DIRECTION ( 'NONE',  ( 0.000000000000000000, 1.000000000000000000, 0.000000000000000000 ) ) ;
#20907=APPLICATION_CONTEXT ( 'automotive_design' ) ;
#20910=DIRECTION ( 'NONE',  ( 0.000000000000000000, 1.000000000000000000, 0.000000000000000000 ) ) ;
#20915=CARTESIAN_POINT ( 'NONE',  ( 1.268730000000000135, 8.334374999999999645, -88.70972349879099283 ) ) ;
#20916=PLANE ( 'NONE',  #6409 ) ;
#20938=CIRCLE ( 'NONE', #9634, 3.175000000000000711 ) ;
#20941=DIRECTION ( 'NONE',  ( 0.8334497143791951279, 0.000000000000000000, 0.5525953072558960066 ) ) ;
#20949=DIRECTION ( 'NONE',  ( 0.000000000000000000, 1.000000000000000000, 0.000000000000000000 ) ) ;
#20953=ORIENTED_EDGE ( 'NONE', *, *, #13437, .T. ) ;
#20961=CARTESIAN_POINT ( 'NONE',  ( 1.776310917873034523, 8.950320134663451555, 8.723978618964752130 ) ) ;
#20962=ORIENTED_EDGE ( 'NONE', *, *, #7376, .F. ) ;
#20965=EDGE_CURVE ( 'NONE', #15944, #8589, #14064, .T. ) ;
#20967=ORIENTED_EDGE ( 'NONE', *, *, #16898, .T. ) ;
#20971=VECTOR ( 'NONE', #1111, 1000.000000000000227 ) ;
#20972=DIRECTION ( 'NONE',  ( 0.000000000000000000, -1.000000000000000000, 0.000000000000000000 ) ) ;
#20976=LINE ( 'NONE', #2294, #3813 ) ;
#20977=ORIENTED_EDGE ( 'NONE', *, *, #289, .F. ) ;
#20980=DIRECTION ( 'NONE',  ( 0.000000000000000000, 1.000000000000000000, 0.000000000000000000 ) ) ;
#20983=ADVANCED_FACE ( 'NONE', ( #20770, #17473 ), #19230, .T. ) ;
#20984=VERTEX_POINT ( 'NONE', #5751 ) ;
#20988=VERTEX_POINT ( 'NONE', #16050 ) ;
#20995=DIRECTION ( 'NONE',  ( -0.9579671649362034858, 0.000000000000000000, 0.2868778675745010109 ) ) ;
#20998=ORIENTED_EDGE ( 'NONE', *, *, #20702, .T. ) ;
#21011=ORIENTED_EDGE ( 'NONE', *, *, #7025, .T. ) ;
#21018=EDGE_CURVE ( 'NONE', #13089, #11451, #4346, .T. ) ;
#21019=LINE ( 'NONE', #2226, #14271 ) ;
#21025=DIRECTION ( 'NONE',  ( 0.000000000000000000, 0.000000000000000000, 1.000000000000000000 ) ) ;
#21048=CARTESIAN_POINT ( 'NONE',  ( 54.36523883999320361, 74.97070807199999365, -30.28170612544299800 ) ) ;
#21056=LINE ( 'NONE', #13009, #11989 ) ;
#21060=VERTEX_POINT ( 'NONE', #978 ) ;
#21065=DIRECTION ( 'NONE',  ( 0.000000000000000000, 1.000000000000000000, 0.000000000000000000 ) ) ;
#21067=ORIENTED_EDGE ( 'NONE', *, *, #9240, .F. ) ;
#21075=LINE ( 'NONE', #9134, #8035 ) ;
#21077=EDGE_LOOP ( 'NONE', ( #17230, #6403, #21686, #10379 ) ) ;
#21089=ADVANCED_FACE ( 'NONE', ( #2618 ), #9238, .T. ) ;
#21090=LINE ( 'NONE', #7511, #19810 ) ;
#21108=ORIENTED_EDGE ( 'NONE', *, *, #6110, .T. ) ;
#21109=LINE ( 'NONE', #5761, #21203 ) ;
#21112=LINE ( 'NONE', #9396, #8384 ) ;
#21123=CARTESIAN_POINT ( 'NONE',  ( -1.345424459097947834, 12.30439499999999953, 2.648158502653860324 ) ) ;
#21134=CARTESIAN_POINT ( 'NONE',  ( 22.60253186962359706, 0.7628563159022999640, 10.29585832510018051 ) ) ;
#21138=VECTOR ( 'NONE', #812, 1000.000000000000000 ) ;
#21139=DIRECTION ( 'NONE',  ( -0.000000000000000000, 1.000000000000000000, 0.000000000000000000 ) ) ;
#21152=DIRECTION ( 'NONE',  ( 0.2868778675745011220, 0.000000000000000000, 0.9579671649362033747 ) ) ;
#21158=ORIENTED_EDGE ( 'NONE', *, *, #19425, .T. ) ;
#21185=DIRECTION ( 'NONE',  ( 1.000000000000000000, 0.000000000000000000, 0.000000000000000000 ) ) ;
#21203=VECTOR ( 'NONE', #4103, 1000.000000000000114 ) ;
#21210=ORIENTED_EDGE ( 'NONE', *, *, #735, .T. ) ;
#21213=DIRECTION ( 'NONE',  ( 0.000000000000000000, 0.000000000000000000, 1.000000000000000000 ) ) ;
#21223=AXIS2_PLACEMENT_3D ( 'NONE', #205, #13711, #13823 ) ;
#21231=DIRECTION ( 'NONE',  ( 1.000000000000000000, 0.000000000000000000, 0.000000000000000000 ) ) ;
#21235=CARTESIAN_POINT ( 'NONE',  ( 54.51779242482700027, 1.984375000000000000, -30.64740209392260084 ) ) ;
#21238=FACE_BOUND ( 'NONE', #7583, .T. ) ;
#21241=ORIENTED_EDGE ( 'NONE', *, *, #6206, .T. ) ;
#21243=AXIS2_PLACEMENT_3D ( 'NONE', #2237, #9305, #19585 ) ;
#21247=CARTESIAN_POINT ( 'NONE',  ( 24.76323281030605017, 0.9575987068668280200, 10.42990517843087872 ) ) ;
#21256=CARTESIAN_POINT ( 'NONE',  ( 67.40134256979101224, 30.56064500000000095, -13.30734117861468135 ) ) ;
#21267=CARTESIAN_POINT ( 'NONE',  ( 65.51436440461340283, 0.000000000000000000, -12.87863775929475985 ) ) ;
#21268=ORIENTED_EDGE ( 'NONE', *, *, #5199, .F. ) ;
#21272=ORIENTED_EDGE ( 'NONE', *, *, #18905, .F. ) ;
#21280=EDGE_CURVE ( 'NONE', #12822, #218, #18796, .T. ) ;
#21281=CARTESIAN_POINT ( 'NONE',  ( -1.848761088705630051, 9.129395000000000593, 7.884515871828260636 ) ) ;
#21283=CARTESIAN_POINT ( 'NONE',  ( 1.916925818690368377, 8.800110775149704523, 8.731250000000001066 ) ) ;
#21291=CIRCLE ( 'NONE', #19547, 0.3962400000000008138 ) ;
#21294=CARTESIAN_POINT ( 'NONE',  ( 49.41235866845560309, 1.984375000000000000, -26.78690084448080100 ) ) ;
#21297=ORIENTED_EDGE ( 'NONE', *, *, #2262, .F. ) ;
#21300=FACE_OUTER_BOUND ( 'NONE', #710, .T. ) ;
#21305=ORIENTED_EDGE ( 'NONE', *, *, #15466, .T. ) ;
#21306=EDGE_CURVE ( 'NONE', #21868, #19865, #9966, .T. ) ;
#21311=VECTOR ( 'NONE', #19323, 1000.000000000000000 ) ;
#21312=CARTESIAN_POINT ( 'NONE',  ( 6.585898268469219552, 30.56064500000000095, 4.694966092919240275 ) ) ;
#21326=CARTESIAN_POINT ( 'NONE',  ( -29.36874999999999858, 30.56064500000000095, 8.335010000000000474 ) ) ;
#21351=CARTESIAN_POINT ( 'NONE',  ( 29.02375794721179858, 1.691909351835945152, 10.69422218668175972 ) ) ;
#21352=EDGE_CURVE ( 'NONE', #14925, #16536, #18940, .T. ) ;
#21355=CARTESIAN_POINT ( 'NONE',  ( -29.36874999999999858, 32.54502000000000095, 8.731885000000000119 ) ) ;
#21359=FACE_OUTER_BOUND ( 'NONE', #13113, .T. ) ;
#21361=DIRECTION ( 'NONE',  ( 0.000000000000000000, 1.000000000000000000, 0.000000000000000000 ) ) ;
#21370=CARTESIAN_POINT ( 'NONE',  ( 28.97711086133420366, 0.000000000000000000, -10.31874999999999964 ) ) ;
#21402=LINE ( 'NONE', #13029, #1451 ) ;
#21403=ORIENTED_EDGE ( 'NONE', *, *, #6553, .F. ) ;
#21408=LINE ( 'NONE', #7928, #3927 ) ;
#21417=EDGE_CURVE ( 'NONE', #6460, #19865, #15992, .T. ) ;
#21423=EDGE_CURVE ( 'NONE', #21532, #2434, #2923, .T. ) ;
#21437=LINE ( 'NONE', #10154, #9546 ) ;
#21439=VECTOR ( 'NONE', #4069, 1000.000000000000000 ) ;
#21441=DIRECTION ( 'NONE',  ( 0.000000000000000000, 1.000000000000000000, 0.000000000000000000 ) ) ;
#21447=ORIENTED_EDGE ( 'NONE', *, *, #15817, .F. ) ;
#21457=CARTESIAN_POINT ( 'NONE',  ( 28.48640205779059897, 1.520289674025695037, 10.66088537228617916 ) ) ;
#21459=AXIS2_PLACEMENT_3D ( 'NONE', #16980, #65, #18857 ) ;
#21463=SURFACE_STYLE_FILL_AREA ( #14757 ) ;
#21464=SHAPE_REPRESENTATION ( 'Ratchet Main Fixed Frame', ( #2234 ), #16895 ) ;
#21469=DIRECTION ( 'NONE',  ( -1.000000000000000000, 0.000000000000000000, 0.000000000000000000 ) ) ;
#21495=CARTESIAN_POINT ( 'NONE',  ( -2.256261688646920227, 22.62314500000000095, -0.3933872460174320240 ) ) ;
#21498=ORIENTED_EDGE ( 'NONE', *, *, #1644, .T. ) ;
#21503=EDGE_CURVE ( 'NONE', #2212, #5739, #16204, .T. ) ;
#21510=ORIENTED_EDGE ( 'NONE', *, *, #19050, .T. ) ;
#21512=CIRCLE ( 'NONE', #3510, 25.00312500000000426 ) ;
#21513=CARTESIAN_POINT ( 'NONE',  ( 70.64340948846358970, 32.54502000000000095, -10.93409647675949969 ) ) ;
#21532=VERTEX_POINT ( 'NONE', #6328 ) ;
#21536=CYLINDRICAL_SURFACE ( 'NONE', #10189, 25.00312499999999361 ) ;
#21541=AXIS2_PLACEMENT_3D ( 'NONE', #19127, #3997, #13629 ) ;
#21542=LINE ( 'NONE', #19987, #8021 ) ;
#21546=DIRECTION ( 'NONE',  ( -0.9999999999672709583, 8.090614674031770259E-06, -1.618640899075949903E-09 ) ) ;
#21562=ORIENTED_EDGE ( 'NONE', *, *, #14486, .F. ) ;
#21567=CARTESIAN_POINT ( 'NONE',  ( 2.063750000000000195, 30.16440499999999858, 8.731249999999999289 ) ) ;
#21568=VERTEX_POINT ( 'NONE', #4361 ) ;
#21571=ORIENTED_EDGE ( 'NONE', *, *, #12516, .F. ) ;
#21572=CIRCLE ( 'NONE', #18742, 0.7950200000000003930 ) ;
#21580=PLANE ( 'NONE',  #15014 ) ;
#21582=DIRECTION ( 'NONE',  ( 1.000000000000000000, 0.000000000000000000, 0.000000000000000000 ) ) ;
#21590=DIRECTION ( 'NONE',  ( 0.000000000000000000, 1.000000000000000000, 0.000000000000000000 ) ) ;
#21606=ORIENTED_EDGE ( 'NONE', *, *, #4822, .T. ) ;
#21607=( NAMED_UNIT ( * ) SI_UNIT ( $, .STERADIAN. ) SOLID_ANGLE_UNIT ( ) );
#21622=DIRECTION ( 'NONE',  ( 0.000000000000000000, 1.000000000000000000, 0.000000000000000000 ) ) ;
#21628=ORIENTED_EDGE ( 'NONE', *, *, #17583, .T. ) ;
#21640=FACE_OUTER_BOUND ( 'NONE', #3609, .T. ) ;
#21641=ORIENTED_EDGE ( 'NONE', *, *, #2922, .T. ) ;
#21653=EDGE_CURVE ( 'NONE', #4933, #10689, #2221, .T. ) ;
#21654=CARTESIAN_POINT ( 'NONE',  ( 46.03750000000000142, 0.000000000000000000, -10.31874999999999964 ) ) ;
#21655=AXIS2_PLACEMENT_3D ( 'NONE', #17852, #2699, #9430 ) ;
#21662=LINE ( 'NONE', #16800, #8849 ) ;
#21663=EDGE_CURVE ( 'NONE', #2434, #2822, #16831, .T. ) ;
#21666=EDGE_CURVE ( 'NONE', #4834, #6050, #14256, .T. ) ;
#21686=ORIENTED_EDGE ( 'NONE', *, *, #2770, .T. ) ;
#21688=EDGE_CURVE ( 'NONE', #14216, #7283, #20938, .T. ) ;
#21694=DIRECTION ( 'NONE',  ( 0.000000000000000000, 0.000000000000000000, 1.000000000000000000 ) ) ;
#21701=CARTESIAN_POINT ( 'NONE',  ( -3.246390552019219999, 20.24316500000000119, 3.217431771123079987 ) ) ;
#21702=CARTESIAN_POINT ( 'NONE',  ( 29.36887348155339694, 1.984374998761125219, 10.71562877576799977 ) ) ;
#21706=EDGE_CURVE ( 'NONE', #16212, #9547, #2588, .T. ) ;
#21708=CARTESIAN_POINT ( 'NONE',  ( 70.64340948846358970, 30.56064500000000095, -10.93409647675949969 ) ) ;
#21712=FACE_OUTER_BOUND ( 'NONE', #1445, .T. ) ;
#21729=LINE ( 'NONE', #6583, #9915 ) ;
#21738=DIRECTION ( 'NONE',  ( 0.9980811434661737147, 0.000000000000000000, 0.06191955310929838502 ) ) ;
#21746=ORIENTED_EDGE ( 'NONE', *, *, #7539, .T. ) ;
#21752=DIRECTION ( 'NONE',  ( 0.000000000000000000, 0.000000000000000000, -1.000000000000000000 ) ) ;
#21758=FACE_OUTER_BOUND ( 'NONE', #13761, .T. ) ;
#21759=DIRECTION ( 'NONE',  ( 1.000000000000000000, 0.000000000000000000, 0.000000000000000000 ) ) ;
#21761=VERTEX_POINT ( 'NONE', #6556 ) ;
#21764=ORIENTED_EDGE ( 'NONE', *, *, #8002, .T. ) ;
#21767=VECTOR ( 'NONE', #141, 1000.000000000000000 ) ;
#21779=EDGE_CURVE ( 'NONE', #13475, #17862, #11065, .T. ) ;
#21782=CARTESIAN_POINT ( 'NONE',  ( 65.64431122251959039, 32.54502000000000095, -11.29787305743958115 ) ) ;
#21783=DIRECTION ( 'NONE',  ( 0.000000000000000000, 1.000000000000000000, 0.000000000000000000 ) ) ;
#21785=DIRECTION ( 'NONE',  ( 0.000000000000000000, 1.000000000000000000, 0.000000000000000000 ) ) ;
#21789=EDGE_LOOP ( 'NONE', ( #4855, #642, #11644, #17445 ) ) ;
#21793=DIRECTION ( 'NONE',  ( 0.000000000000000000, 0.000000000000000000, 1.000000000000000000 ) ) ;
#21794=AXIS2_PLACEMENT_3D ( 'NONE', #12245, #8691, #7036 ) ;
#21795=DIRECTION ( 'NONE',  ( 1.000000000000000000, 0.000000000000000000, 0.000000000000000000 ) ) ;
#21802=DIRECTION ( 'NONE',  ( 0.000000000000000000, 0.000000000000000000, -1.000000000000000000 ) ) ;
#21804=CARTESIAN_POINT ( 'NONE',  ( 29.36874999999999858, 22.62187499999999929, 10.71562499999999929 ) ) ;
#21807=CIRCLE ( 'NONE', #5205, 1.983740000000000059 ) ;
#21810=LINE ( 'NONE', #5121, #5177 ) ;
#21811=EDGE_CURVE ( 'NONE', #8805, #10798, #10699, .T. ) ;
#21812=ORIENTED_EDGE ( 'NONE', *, *, #16068, .F. ) ;
#21814=DIRECTION ( 'NONE',  ( 0.000000000000000000, -1.000000000000000000, 0.000000000000000000 ) ) ;
#21819=VERTEX_POINT ( 'NONE', #10852 ) ;
#21821=CARTESIAN_POINT ( 'NONE',  ( -29.36874999999999858, 30.16440499999999858, 8.731249999999999289 ) ) ;
#21836=FACE_OUTER_BOUND ( 'NONE', #5480, .T. ) ;
#21846=DIRECTION ( 'NONE',  ( 1.000000000000000000, 0.000000000000000000, 0.000000000000000000 ) ) ;
#21849=VERTEX_POINT ( 'NONE', #12297 ) ;
#21850=AXIS2_PLACEMENT_3D ( 'NONE', #14533, #12761, #2692 ) ;
#21856=AXIS2_PLACEMENT_3D ( 'NONE', #5491, #10144, #18975 ) ;
#21863=DIRECTION ( 'NONE',  ( 0.8334497143791951279, 0.000000000000000000, 0.5525953072558960066 ) ) ;
#21864=DIRECTION ( 'NONE',  ( 0.000000000000000000, 1.000000000000000000, 0.000000000000000000 ) ) ;
#21866=VECTOR ( 'NONE', #1572, 1000.000000000000114 ) ;
#21868=VERTEX_POINT ( 'NONE', #19254 ) ;
#21874=DIRECTION ( 'NONE',  ( 0.000000000000000000, 1.000000000000000000, 0.000000000000000000 ) ) ;
#21875=ORIENTED_EDGE ( 'NONE', *, *, #3771, .F. ) ;
#21881=CYLINDRICAL_SURFACE ( 'NONE', #12552, 0.3962400000000008138 ) ;
ENDSEC;
END-ISO-10303-21;
